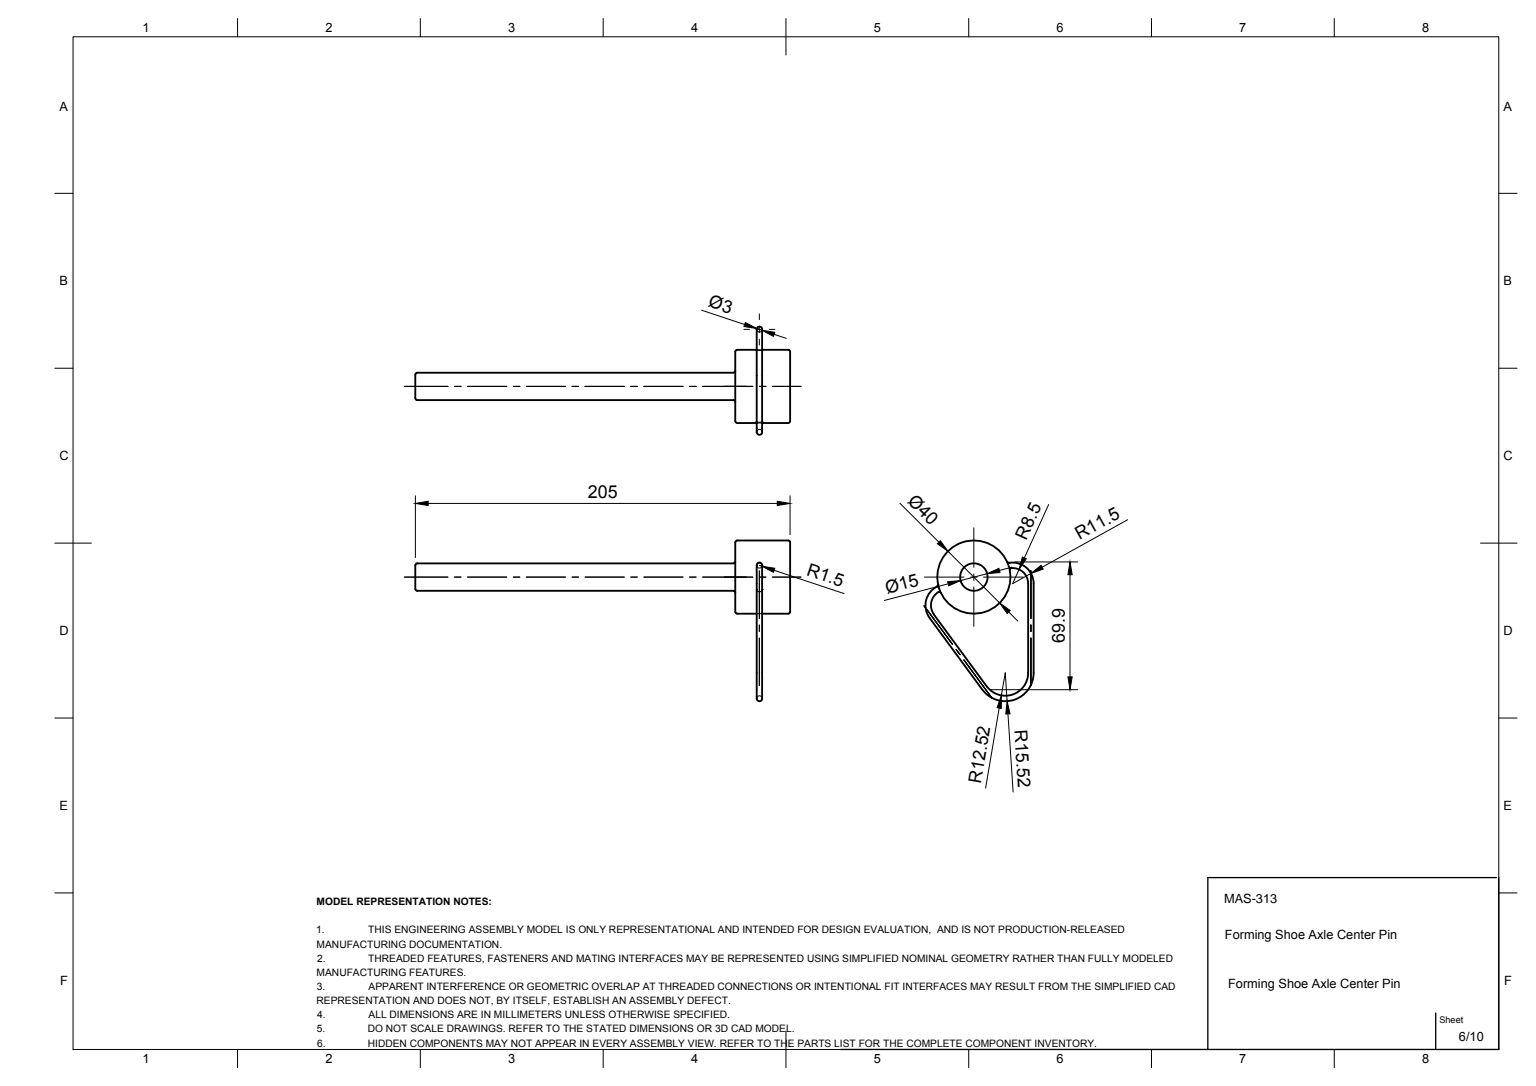
ISO-10303-21;
HEADER;
FILE_DESCRIPTION (('STEP AP214'),
    '1' );
FILE_NAME ('Forming Shoe Axle Center Pin.step',
    '2026-10-06T09:36:00',
    ( '' ),
    ( '' ),
    'SwSTEP 2.0',
    'SolidWorks 2025',
    '' );
FILE_SCHEMA (( 'AUTOMOTIVE_DESIGN' ));
ENDSEC;

DATA;
#20=VERTEX_POINT ( 'NONE', #8026 ) ;
#27=AXIS2_PLACEMENT_3D ( 'NONE', #9687, #6908, #2335 ) ;
#30=CARTESIAN_POINT ( 'NONE',  ( 19.97706055966621008, 179.9215598820742628, -126.1361639878079757 ) ) ;
#44=CARTESIAN_POINT ( 'NONE',  ( -20.77482174596512010, 180.9926187296579201, -123.5402880645762451 ) ) ;
#47=EDGE_CURVE ( 'NONE', #6610, #12185, #4189, .T. ) ;
#58=ORIENTED_EDGE ( 'NONE', *, *, #10485, .F. ) ;
#78=CARTESIAN_POINT ( 'NONE',  ( 19.99739293773369653, 178.7258229095291426, -125.0390604444466902 ) ) ;
#93=EDGE_CURVE ( 'NONE', #7054, #9028, #4139, .T. ) ;
#99=FACE_OUTER_BOUND ( 'NONE', #2484, .T. ) ;
#100=CARTESIAN_POINT ( 'NONE',  ( -19.99217429592516737, 178.8549194765174946, -125.3522826812394584 ) ) ;
#108=CARTESIAN_POINT ( 'NONE',  ( 19.97032670689476674, 177.8811654734197134, -125.7875625598146883 ) ) ;
#126=CARTESIAN_POINT ( 'NONE',  ( 19.97657209060318806, 179.2792238463859746, -123.5006916350263282 ) ) ;
#127=CARTESIAN_POINT ( 'NONE',  ( -21.00467209899894172, 181.7165653707129422, -124.9111601018296795 ) ) ;
#151=CARTESIAN_POINT ( 'NONE',  ( -19.98114923013653765, 179.3963068953591176, -125.9321215961336975 ) ) ;
#154=VERTEX_POINT ( 'NONE', #2390 ) ;
#156=AXIS2_PLACEMENT_3D ( 'NONE', #6549, #9206, #9335 ) ;
#159=DIRECTION ( 'NONE',  ( -1.186840563529527301E-16, 1.000000000000000000, -0.000000000000000000 ) ) ;
#162=CARTESIAN_POINT ( 'NONE',  ( -20.82968904857387216, 181.3053215700974192, -123.7910769712144798 ) ) ;
#176=AXIS2_PLACEMENT_3D ( 'NONE', #10566, #11560, #2167 ) ;
#213=VECTOR ( 'NONE', #11605, 1000.000000000000000 ) ;
#221=DIRECTION ( 'NONE',  ( -1.000000000000000000, 0.000000000000000000, 0.000000000000000000 ) ) ;
#222=CARTESIAN_POINT ( 'NONE',  ( 19.92179295512113057, 178.7027072646551744, -122.9085123094865537 ) ) ;
#236=DIRECTION ( 'NONE',  ( -0.000000000000000000, -1.000000000000000000, -1.757987137413040192E-14 ) ) ;
#248=FACE_OUTER_BOUND ( 'NONE', #11895, .T. ) ;
#255=CARTESIAN_POINT ( 'NONE',  ( 20.99826841500651753, 178.6919330321067036, -124.8534679218782770 ) ) ;
#262=DIRECTION ( 'NONE',  ( 1.186840563529527301E-16, -1.000000000000000000, 0.000000000000000000 ) ) ;
#274=CARTESIAN_POINT ( 'NONE',  ( -21.06063637301984670, 178.9270029669538360, -125.6999331669520501 ) ) ;
#275=CIRCLE ( 'NONE', #3413, 1.000000000000001110 ) ;
#289=ORIENTED_EDGE ( 'NONE', *, *, #5265, .F. ) ;
#292=CARTESIAN_POINT ( 'NONE',  ( -13.32222501832919193, 180.2041921146325762, -184.1652315311841051 ) ) ;
#295=CARTESIAN_POINT ( 'NONE',  ( -7.499999999999979572, -6.999999999999979572, -124.6807709998038405 ) ) ;
#303=DIRECTION ( 'NONE',  ( -1.186840563529527301E-16, 1.000000000000000000, -0.000000000000000000 ) ) ;
#307=EDGE_CURVE ( 'NONE', #1954, #154, #9065, .T. ) ;
#332=AXIS2_PLACEMENT_3D ( 'NONE', #843, #8325, #8259 ) ;
#337=CARTESIAN_POINT ( 'NONE',  ( 19.00000000000000000, 197.0000000000000000, -124.6807709998038405 ) ) ;
#372=DIRECTION ( 'NONE',  ( 0.000000000000000000, -1.000000000000000000, -1.850371707708592551E-14 ) ) ;
#377=EDGE_LOOP ( 'NONE', ( #4540, #1681, #1210, #5686, #11186, #2942, #6085, #5745, #3833, #8762 ) ) ;
#406=PRODUCT_DEFINITION ( 'UNKNOWN', '', #11578, #8636 ) ;
#416=CARTESIAN_POINT ( 'NONE',  ( 19.96510381999703654, 179.6655525025668680, -123.2864411696423019 ) ) ;
#423=AXIS2_PLACEMENT_3D ( 'NONE', #2783, #4705, #7030 ) ;
#446=ADVANCED_FACE ( 'NONE', ( #2952 ), #990, .T. ) ;
#447=ORIENTED_EDGE ( 'NONE', *, *, #3448, .T. ) ;
#457=CARTESIAN_POINT ( 'NONE',  ( -20.81528965651789420, 181.2703058956580264, -123.7202784472551258 ) ) ;
#459=CARTESIAN_POINT ( 'NONE',  ( 19.83353877203827764, 180.5116607636902302, -127.2558091114354966 ) ) ;
#460=CARTESIAN_POINT ( 'NONE',  ( 19.88442870626286307, 179.4513098237186455, -122.5333155736647655 ) ) ;
#462=VECTOR ( 'NONE', #11784, 1000.000000000000000 ) ;
#465=CARTESIAN_POINT ( 'NONE',  ( 20.00000000000000000, 197.0000000000000000, -124.6807709998038405 ) ) ;
#476=DIRECTION ( 'NONE',  ( 0.000000000000000000, 1.632680918566399772E-14, -1.000000000000000000 ) ) ;
#490=ADVANCED_FACE ( 'NONE', ( #99 ), #10651, .T. ) ;
#491=CARTESIAN_POINT ( 'NONE',  ( -20.90635653397698590, 181.5182364730088125, -122.6997973820476489 ) ) ;
#497=CARTESIAN_POINT ( 'NONE',  ( -19.97664783916611952, 180.3484222408143296, -126.1556734819005925 ) ) ;
#505=VERTEX_POINT ( 'NONE', #2202 ) ;
#513=CARTESIAN_POINT ( 'NONE',  ( -19.99999999999999645, 177.7115707886035807, -124.6807709997916334 ) ) ;
#520=CARTESIAN_POINT ( 'NONE',  ( 7.750278301654327992E-16, 197.0000000000000000, -124.6807709998038405 ) ) ;
#527=CARTESIAN_POINT ( 'NONE',  ( 19.83120603885254951, 180.1820437873792287, -127.2737130629590041 ) ) ;
#539=FACE_OUTER_BOUND ( 'NONE', #6413, .T. ) ;
#547=CARTESIAN_POINT ( 'NONE',  ( 19.96803729195536548, 180.8767316306619932, -123.3312649246138051 ) ) ;
#552=CIRCLE ( 'NONE', #6873, 0.9999999999999986677 ) ;
#556=CARTESIAN_POINT ( 'NONE',  ( 19.03136272649511085, 180.2041921146316668, -134.6807709998038547 ) ) ;
#559=VERTEX_POINT ( 'NONE', #337 ) ;
#567=CARTESIAN_POINT ( 'NONE',  ( -19.85757705203717549, 179.1763491573645979, -127.0639759997010714 ) ) ;
#569=VERTEX_POINT ( 'NONE', #9980 ) ;
#573=ORIENTED_EDGE ( 'NONE', *, *, #3270, .F. ) ;
#574=B_SPLINE_CURVE_WITH_KNOTS ( 'NONE', 3,
 ( #6859, #1412, #10623, #7851, #11679, #11625, #6974, #2280, #11742, #8936, #3144, #10680, #1355, #2218 ),
 .UNSPECIFIED., .F., .F.,
 ( 4, 2, 2, 2, 2, 2, 4 ),
 ( 0.005787645201702338975, 0.006295307287268509314, 0.006802969372834680520, 0.007818293543967111403, 0.008833617715099544021, 0.009341279800665706554, 0.009848941886231869086 ),
 .UNSPECIFIED. ) ;
#583=CARTESIAN_POINT ( 'NONE',  ( -7.500000000000004441, 197.0000000000000000, -124.6807709998038405 ) ) ;
#585=DIRECTION ( 'NONE',  ( -1.186840563529527301E-16, 1.000000000000000000, -0.000000000000000000 ) ) ;
#587=CARTESIAN_POINT ( 'NONE',  ( -21.05657978152897769, 178.8587358379057548, -125.5860039436037567 ) ) ;
#588=( NAMED_UNIT ( * ) SI_UNIT ( $, .STERADIAN. ) SOLID_ANGLE_UNIT ( ) );
#598=B_SPLINE_CURVE_WITH_KNOTS ( 'NONE', 3,
 ( #6314, #1680, #9286, #7245, #826, #4597, #888, #8437, #5439, #11267, #7428, #8371, #4716, #2601, #5375, #11011, #757, #9151, #3650, #4535 ),
 .UNSPECIFIED., .F., .F.,
 ( 4, 2, 2, 2, 2, 2, 2, 2, 2, 4 ),
 ( 0.009933187713138447172, 0.01060625352217340472, 0.01094278642669084187, 0.01127931933120827901, 0.01195238514024315329, 0.01262545094927802758, 0.01329851675831290360, 0.01397158256734777788, 0.01464464837638265217, 0.01531771418541752645 ),
 .UNSPECIFIED. ) ;
#608=CARTESIAN_POINT ( 'NONE',  ( 20.00048861043547177, 181.7193014332009113, -124.6844417253709025 ) ) ;
#610=CARTESIAN_POINT ( 'NONE',  ( 19.89275938512204078, 181.1945314693525972, -122.6057198881955941 ) ) ;
#611=AXIS2_PLACEMENT_3D ( 'NONE', #3672, #6457, #11093 ) ;
#612=CARTESIAN_POINT ( 'NONE',  ( -19.97551221440360436, 178.0138700112367758, -123.6762749394707441 ) ) ;
#616=EDGE_CURVE ( 'NONE', #4019, #1329, #9737, .T. ) ;
#618=DIRECTION ( 'NONE',  ( -0.000000000000000000, -1.000000000000000000, -1.757987137413040192E-14 ) ) ;
#630=CARTESIAN_POINT ( 'NONE',  ( -21.06735260060543879, 180.9331586078316150, -126.2486801514333905 ) ) ;
#636=DIRECTION ( 'NONE',  ( -1.186840563529527301E-16, 1.000000000000000000, -0.000000000000000000 ) ) ;
#646=CIRCLE ( 'NONE', #1249, 11.50000000000003730 ) ;
#651=EDGE_CURVE ( 'NONE', #6732, #6027, #3151, .T. ) ;
#659=CARTESIAN_POINT ( 'NONE',  ( -20.73244433232022033, 180.6366558386295935, -123.3579215951269248 ) ) ;
#674=CARTESIAN_POINT ( 'NONE',  ( 19.99815408692506580, 181.6905235212389869, -124.9672463342703566 ) ) ;
#677=CARTESIAN_POINT ( 'NONE',  ( -19.83634048512597658, 179.7265707582143079, -127.2348386560517781 ) ) ;
#692=ADVANCED_FACE ( 'NONE', ( #4300 ), #5147, .T. ) ;
#695=ORIENTED_EDGE ( 'NONE', *, *, #8586, .T. ) ;
#712=ORIENTED_EDGE ( 'NONE', *, *, #11302, .F. ) ;
#713=CARTESIAN_POINT ( 'NONE',  ( -21.06729583384051097, 179.4139655881280078, -126.1965993184190040 ) ) ;
#737=ORIENTED_EDGE ( 'NONE', *, *, #10086, .T. ) ;
#740=EDGE_CURVE ( 'NONE', #4344, #2611, #2200, .T. ) ;
#750=CARTESIAN_POINT ( 'NONE',  ( -20.00000000000000000, 197.0000000000000000, -124.6807709998038405 ) ) ;
#757=CARTESIAN_POINT ( 'NONE',  ( 19.83551131833741010, 179.7633983601342038, -127.2411838750873727 ) ) ;
#761=LINE ( 'NONE', #10215, #10128 ) ;
#765=ORIENTED_EDGE ( 'NONE', *, *, #11667, .F. ) ;
#768=CARTESIAN_POINT ( 'NONE',  ( -19.87519864879851994, 178.8871479037923393, -126.9115732480538838 ) ) ;
#770=( BOUNDED_SURFACE ( )  B_SPLINE_SURFACE ( 3, 2, ( 
 ( #7122, #2418, #6198 ),
 ( #9783, #2308, #9966 ),
 ( #6078, #8742, #659 ),
 ( #4630, #9252, #12035 ),
 ( #4435, #11044, #2570 ),
 ( #795, #4563, #923 ),
 ( #8340, #4499, #8410 ),
 ( #2770, #1648, #11178 ),
 ( #8211, #9122, #11245 ),
 ( #11973, #3548, #3689 ),
 ( #12104, #12172, #2702 ),
 ( #5409, #9317, #7337 ),
 ( #3613, #862, #7404 ),
 ( #6473, #11109, #3491 ),
 ( #7276, #6341, #10116 ),
 ( #10247, #2631, #1842 ),
 ( #6410, #1782, #7465 ),
 ( #5545, #6534, #10302 ),
 ( #5606, #9383, #4696 ),
 ( #10608, #11354, #7646 ),
 ( #3810, #10544, #8576 ),
 ( #9441, #10489, #4918 ),
 ( #8700, #100, #978 ),
 ( #3874, #9680, #9559 ),
 ( #7582, #2953, #274 ),
 ( #3998, #6715, #2022 ),
 ( #1105, #1218, #8639 ),
 ( #5911, #2146, #2091 ),
 ( #8758, #151, #9619 ),
 ( #7766, #4065, #5460 ) ),
 .UNSPECIFIED., .F., .F., .F. ) 
 B_SPLINE_SURFACE_WITH_KNOTS ( ( 4, 2, 2, 2, 2, 2, 2, 2, 2, 2, 2, 2, 2, 2, 4 ),
 ( 3, 3 ),
 ( 0.007888614278243437361, 0.008874691063023869633, 0.009367729455414086637, 0.009860767847804301905, 0.01035380624019451891, 0.01084684463258473591, 0.01133988302497495118, 0.01183292141736516818, 0.01281899820214560046, 0.01331203659453581746, 0.01380507498692603446, 0.01429811337931624973, 0.01479115177170646674, 0.01528419016409668374, 0.01577722855648689901 ),
 ( 0.000000000000000000, 1.000000000000000000 ),
 .UNSPECIFIED. ) 
 GEOMETRIC_REPRESENTATION_ITEM ( )  RATIONAL_B_SPLINE_SURFACE ( (
 ( 1.000000000000000000, 0.7778924984312529656, 1.000000000000000000),
 ( 1.000000000000000000, 0.7847112435279847142, 1.000000000000000000),
 ( 1.000000000000000000, 0.7894485421771765266, 1.000000000000000000),
 ( 1.000000000000000000, 0.7926414855251958658, 1.000000000000000000),
 ( 1.000000000000000000, 0.7930469064958857173, 1.000000000000000000),
 ( 1.000000000000000000, 0.7925074991235926403, 1.000000000000000000),
 ( 1.000000000000000000, 0.7915770372355392936, 1.000000000000000000),
 ( 1.000000000000000000, 0.7883898363194743464, 1.000000000000000000),
 ( 1.000000000000000000, 0.7861853387937841608, 1.000000000000000000),
 ( 1.000000000000000000, 0.7806815604416567078, 1.000000000000000000),
 ( 1.000000000000000000, 0.7773361016722152295, 1.000000000000000000),
 ( 1.000000000000000000, 0.7698701636707948603, 1.000000000000000000),
 ( 1.000000000000000000, 0.7657526702509508398, 1.000000000000000000),
 ( 1.000000000000000000, 0.7568812398704235500, 1.000000000000000000),
 ( 1.000000000000000000, 0.7521322257284934754, 1.000000000000000000),
 ( 1.000000000000000000, 0.7377220824064392168, 1.000000000000000000),
 ( 1.000000000000000000, 0.7275566802060602356, 1.000000000000000000),
 ( 1.000000000000000000, 0.7135779984947178134, 1.000000000000000000),
 ( 1.000000000000000000, 0.7090467312072497030, 1.000000000000000000),
 ( 1.000000000000000000, 0.7006183237057392876, 1.000000000000000000),
 ( 1.000000000000000000, 0.6967528866742972449, 1.000000000000000000),
 ( 1.000000000000000000, 0.6897151435478420245, 1.000000000000000000),
 ( 1.000000000000000000, 0.6865208713865151857, 1.000000000000000000),
 ( 1.000000000000000000, 0.6810351634549236532, 1.000000000000000000),
 ( 1.000000000000000000, 0.6787116622188523740, 1.000000000000000000),
 ( 1.000000000000000000, 0.6747765002012137137, 1.000000000000000000),
 ( 1.000000000000000000, 0.6731806124592021323, 1.000000000000000000),
 ( 1.000000000000000000, 0.6706618708365198467, 1.000000000000000000),
 ( 1.000000000000000000, 0.6697163794380122104, 1.000000000000000000),
 ( 1.000000000000000000, 0.6689879873414465994, 1.000000000000000000) ) ) 
 REPRESENTATION_ITEM ( '' )  SURFACE ( )  );
#773=CARTESIAN_POINT ( 'NONE',  ( 19.87268743161337170, 178.9255784920988503, -126.9338343023757290 ) ) ;
#780=ORIENTED_EDGE ( 'NONE', *, *, #4037, .T. ) ;
#786=DIRECTION ( 'NONE',  ( -1.000000000000000000, 0.000000000000000000, 0.000000000000000000 ) ) ;
#791=CIRCLE ( 'NONE', #11439, 12.52076803445814690 ) ;
#792=PLANE ( 'NONE',  #6380 ) ;
#795=CARTESIAN_POINT ( 'NONE',  ( -19.87376422533415266, 179.9397883299151601, -122.4372163154974942 ) ) ;
#804=CARTESIAN_POINT ( 'NONE',  ( 21.06240745282767435, 180.2041921146315246, -126.4269926335259413 ) ) ;
#808=CARTESIAN_POINT ( 'NONE',  ( 19.86936981681406778, 181.4590435457396609, -126.9708661016945257 ) ) ;
#822=VERTEX_POINT ( 'NONE', #12019 ) ;
#826=CARTESIAN_POINT ( 'NONE',  ( 19.98066683771208574, 182.6001984525962030, -125.5662099944124748 ) ) ;
#830=CARTESIAN_POINT ( 'NONE',  ( -19.99331759212207515, 182.5955720455716573, -124.1413515841623649 ) ) ;
#839=AXIS2_PLACEMENT_3D ( 'NONE', #11119, #4323, #8349 ) ;
#843=CARTESIAN_POINT ( 'NONE',  ( -19.03136272649511085, 180.2041921146316668, -134.6807709998038547 ) ) ;
#862=CARTESIAN_POINT ( 'NONE',  ( -19.98517529853678809, 179.0632710820790976, -123.7013734869633197 ) ) ;
#870=CARTESIAN_POINT ( 'NONE',  ( 19.99218703114167539, 182.5822718396941582, -124.1010742661679274 ) ) ;
#888=CARTESIAN_POINT ( 'NONE',  ( 19.96426536123311735, 182.4767232793243181, -125.8798892712007245 ) ) ;
#894=CARTESIAN_POINT ( 'NONE',  ( -20.00092085174054546, 181.7296212712162173, -124.7139161294905136 ) ) ;
#909=CARTESIAN_POINT ( 'NONE',  ( 21.04869859328100290, 178.8069441414488097, -125.4530315734257471 ) ) ;
#913=EDGE_CURVE ( 'NONE', #9220, #9416, #3010, .T. ) ;
#914=AXIS2_PLACEMENT_3D ( 'NONE', #2500, #4427, #1515 ) ;
#923=CARTESIAN_POINT ( 'NONE',  ( -20.72096896666972299, 180.0455498438134896, -123.3107784691637079 ) ) ;
#926=CARTESIAN_POINT ( 'NONE',  ( -21.06240745282767080, 180.2041921146517041, -126.4269926335259413 ) ) ;
#927=ORIENTED_EDGE ( 'NONE', *, *, #5402, .T. ) ;
#936=DIRECTION ( 'NONE',  ( -0.000000000000000000, -1.000000000000000000, -1.757987137413040192E-14 ) ) ;
#942=EDGE_LOOP ( 'NONE', ( #4491, #737, #7354, #4686, #5672 ) ) ;
#955=B_SPLINE_CURVE_WITH_KNOTS ( 'NONE', 3,
 ( #11864, #5021, #2525, #4106, #10938, #8230, #9138, #11926, #3379, #10652, #7171, #10998, #5360, #612, #1542, #5303, #3167, #6016 ),
 .UNSPECIFIED., .F., .F.,
 ( 4, 2, 2, 2, 2, 2, 2, 2, 4 ),
 ( 0.007924218878882885106, 0.008564103707084826447, 0.009203988535286766054, 0.009843873363488707395, 0.01048375819169064874, 0.01112364301989258834, 0.01176352784809452968, 0.01240341267629646929, 0.01304329750449841063 ),
 .UNSPECIFIED. ) ;
#968=CARTESIAN_POINT ( 'NONE',  ( 27.10787553788151172, 180.2041921146317520, -137.3302880892914288 ) ) ;
#971=ORIENTED_EDGE ( 'NONE', *, *, #9425, .T. ) ;
#978=CARTESIAN_POINT ( 'NONE',  ( -21.04715153834148467, 178.7974658297258372, -125.4275705862621066 ) ) ;
#980=ORIENTED_EDGE ( 'NONE', *, *, #11838, .T. ) ;
#983=AXIS2_PLACEMENT_3D ( 'NONE', #1406, #8087, #9811 ) ;
#990=TOROIDAL_SURFACE ( 'NONE', #6899, 10.00000000000002487, 1.499999999999998002 ) ;
#1006=CARTESIAN_POINT ( 'NONE',  ( 20.86846003075320866, 178.9597637446144631, -123.9944097082106396 ) ) ;
#1007=EDGE_CURVE ( 'NONE', #6027, #2717, #3007, .T. ) ;
#1009=CARTESIAN_POINT ( 'NONE',  ( -20.00222207760924320, 182.7106143631367559, -124.6033207595390593 ) ) ;
#1015=FACE_OUTER_BOUND ( 'NONE', #7771, .T. ) ;
#1028=ORIENTED_EDGE ( 'NONE', *, *, #10086, .F. ) ;
#1036=EDGE_CURVE ( 'NONE', #7665, #6732, #955, .T. ) ;
#1039=FACE_OUTER_BOUND ( 'NONE', #11944, .T. ) ;
#1040=CARTESIAN_POINT ( 'NONE',  ( 21.06408185580648862, 179.7982817377094591, -126.3732375885690260 ) ) ;
#1052=CARTESIAN_POINT ( 'NONE',  ( -19.03136272649511085, 180.2041921146316668, -134.6807709998038547 ) ) ;
#1054=CARTESIAN_POINT ( 'NONE',  ( 19.94460181908782914, 178.0949482486194597, -126.1813690857228636 ) ) ;
#1057=EDGE_LOOP ( 'NONE', ( #6785, #9431, #1351, #2666, #10669 ) ) ;
#1059=DIRECTION ( 'NONE',  ( -0.3117078928809425831, -5.319854888938806247E-14, 0.9501779778103273122 ) ) ;
#1071=CARTESIAN_POINT ( 'NONE',  ( 19.96762839730446260, 179.5630691651248299, -123.3296266449212766 ) ) ;
#1085=EDGE_LOOP ( 'NONE', ( #10428, #11076, #8480, #3695 ) ) ;
#1105=CARTESIAN_POINT ( 'NONE',  ( -19.91567555516949994, 178.3764997479877650, -126.5185459719826468 ) ) ;
#1106=CARTESIAN_POINT ( 'NONE',  ( 19.03136272649511085, 180.2041921146316668, -134.6807709998038547 ) ) ;
#1126=PRODUCT_DEFINITION_SHAPE ( 'NONE', 'NONE',  #406 ) ;
#1161=FACE_OUTER_BOUND ( 'NONE', #10213, .T. ) ;
#1162=AXIS2_PLACEMENT_3D ( 'NONE', #4182, #1345, #5107 ) ;
#1172=CIRCLE ( 'NONE', #8067, 1.500000000000001332 ) ;
#1187=EDGE_CURVE ( 'NONE', #3899, #2611, #5763, .T. ) ;
#1202=EDGE_LOOP ( 'NONE', ( #3605, #10463 ) ) ;
#1206=CARTESIAN_POINT ( 'NONE',  ( -19.99999999999992184, 182.7057073811386658, -124.7928861707884494 ) ) ;
#1210=ORIENTED_EDGE ( 'NONE', *, *, #1523, .T. ) ;
#1218=CARTESIAN_POINT ( 'NONE',  ( -19.98421530564996473, 179.1834412406901151, -125.7728037431097619 ) ) ;
#1249=AXIS2_PLACEMENT_3D ( 'NONE', #8612, #6689, #6811 ) ;
#1258=EDGE_CURVE ( 'NONE', #4474, #4344, #12188, .T. ) ;
#1261=CARTESIAN_POINT ( 'NONE',  ( -19.99234306063619471, 182.6762740227041206, -125.2450393957101653 ) ) ;
#1283=ORIENTED_EDGE ( 'NONE', *, *, #5915, .F. ) ;
#1299=CIRCLE ( 'NONE', #5225, 19.00000000000000000 ) ;
#1310=CARTESIAN_POINT ( 'NONE',  ( 19.97422267005788044, 181.0592659262004247, -123.4551364493781733 ) ) ;
#1322=CARTESIAN_POINT ( 'NONE',  ( -19.85981914806637860, 181.2821069731401735, -127.0472120087121652 ) ) ;
#1323=FACE_OUTER_BOUND ( 'NONE', #10059, .T. ) ;
#1329=VERTEX_POINT ( 'NONE', #10442 ) ;
#1345=DIRECTION ( 'NONE',  ( 0.3117078928809249860, 1.670400663243698742E-14, -0.9501779778103330854 ) ) ;
#1348=CARTESIAN_POINT ( 'NONE',  ( 19.94418390071693281, 178.3880804771991677, -123.1813497959713004 ) ) ;
#1351=ORIENTED_EDGE ( 'NONE', *, *, #11667, .T. ) ;
#1355=CARTESIAN_POINT ( 'NONE',  ( 21.06813109674855156, 179.2925129078113571, -126.1227452162743674 ) ) ;
#1378=CARTESIAN_POINT ( 'NONE',  ( 20.91518010789754456, 178.8209456716285501, -124.2613132543053638 ) ) ;
#1381=ORIENTED_EDGE ( 'NONE', *, *, #2835, .T. ) ;
#1387=UNCERTAINTY_MEASURE_WITH_UNIT (LENGTH_MEASURE( 1.000000000000000082E-05 ), #8332, 'distance_accuracy_value', 'NONE');
#1397=LINE ( 'NONE', #4245, #462 ) ;
#1406=CARTESIAN_POINT ( 'NONE',  ( 28.53314250459842327, 180.2041921146317236, -137.7978499286132319 ) ) ;
#1412=CARTESIAN_POINT ( 'NONE',  ( 20.71964524312697620, 180.0370539397483185, -123.3053720114571519 ) ) ;
#1413=DIRECTION ( 'NONE',  ( -1.000000000000000000, 0.000000000000000000, 0.000000000000000000 ) ) ;
#1419=CARTESIAN_POINT ( 'NONE',  ( -19.03136272649511085, 180.2041921146316668, -134.6807709998038547 ) ) ;
#1428=DIRECTION ( 'NONE',  ( -1.000000000000000000, 0.000000000000000000, 0.000000000000000000 ) ) ;
#1430=DIRECTION ( 'NONE',  ( -1.000000000000000000, 0.000000000000000000, 0.000000000000000000 ) ) ;
#1448=FACE_OUTER_BOUND ( 'NONE', #11473, .T. ) ;
#1453=CIRCLE ( 'NONE', #4229, 1.500000000000001332 ) ;
#1482=EDGE_LOOP ( 'NONE', ( #2546, #3392, #12236, #9462 ) ) ;
#1498=FACE_OUTER_BOUND ( 'NONE', #3824, .T. ) ;
#1515=DIRECTION ( 'NONE',  ( -1.000000000000000000, 0.000000000000000000, 0.000000000000000000 ) ) ;
#1516=ORIENTED_EDGE ( 'NONE', *, *, #5402, .F. ) ;
#1520=CARTESIAN_POINT ( 'NONE',  ( 19.90865200055593220, 181.4799304009739558, -122.7714319726113104 ) ) ;
#1523=EDGE_CURVE ( 'NONE', #2536, #6732, #761, .T. ) ;
#1541=ADVANCED_FACE ( 'NONE', ( #1498 ), #4158, .F. ) ;
#1542=CARTESIAN_POINT ( 'NONE',  ( -19.98431733801637122, 177.9165942756023640, -123.8639317673912785 ) ) ;
#1543=DIRECTION ( 'NONE',  ( 1.000000000000000000, 1.186840563529527301E-16, 0.000000000000000000 ) ) ;
#1555=CARTESIAN_POINT ( 'NONE',  ( -19.97950307607502296, 180.8737719992032567, -126.0168746971561688 ) ) ;
#1556=DIRECTION ( 'NONE',  ( -0.000000000000000000, -1.000000000000000000, -1.757987137413040192E-14 ) ) ;
#1596=CARTESIAN_POINT ( 'NONE',  ( 19.98721147511798080, 181.3928720024498205, -123.7411646176790327 ) ) ;
#1620=CARTESIAN_POINT ( 'NONE',  ( -19.97661686088444810, 180.0768701897325741, -126.1571822173844453 ) ) ;
#1627=CIRCLE ( 'NONE', #5771, 7.500000000000005329 ) ;
#1645=EDGE_CURVE ( 'NONE', #8550, #1954, #6674, .T. ) ;
#1648=CARTESIAN_POINT ( 'NONE',  ( -19.96447914003645607, 179.6944185909774490, -123.2758706440192213 ) ) ;
#1651=ORIENTED_EDGE ( 'NONE', *, *, #3988, .F. ) ;
#1661=CARTESIAN_POINT ( 'NONE',  ( 19.99452644844618732, 181.5558364952455577, -124.0087194824425865 ) ) ;
#1671=AXIS2_PLACEMENT_3D ( 'NONE', #8007, #9792, #8865 ) ;
#1680=CARTESIAN_POINT ( 'NONE',  ( 19.99999999999986855, 182.7144438187336277, -124.9030158930556667 ) ) ;
#1681=ORIENTED_EDGE ( 'NONE', *, *, #11312, .T. ) ;
#1692=EDGE_CURVE ( 'NONE', #11672, #7759, #8013, .T. ) ;
#1693=CYLINDRICAL_SURFACE ( 'NONE', #8004, 1.500000000000000444 ) ;
#1695=CARTESIAN_POINT ( 'NONE',  ( 21.06714599819344258, 179.1261101450867557, -125.9628648169738625 ) ) ;
#1714=CARTESIAN_POINT ( 'NONE',  ( 19.86348653241994100, 179.0685786869776450, -127.0149889656965740 ) ) ;
#1728=FACE_BOUND ( 'NONE', #8840, .T. ) ;
#1731=CARTESIAN_POINT ( 'NONE',  ( 19.92971727147881467, 178.2306503425758990, -126.3637072540984292 ) ) ;
#1733=CARTESIAN_POINT ( 'NONE',  ( 20.00016885954969226, 181.6903612530189491, -124.3916023546908463 ) ) ;
#1739=CARTESIAN_POINT ( 'NONE',  ( 21.06635469844951558, 179.5529625613920643, -126.2817468820535964 ) ) ;
#1745=TOROIDAL_SURFACE ( 'NONE', #10019, 6.500000000000005329, 1.000000000000000000 ) ;
#1774=DIRECTION ( 'NONE',  ( -1.186840563529527301E-16, 1.000000000000000000, -0.000000000000000000 ) ) ;
#1782=CARTESIAN_POINT ( 'NONE',  ( -20.00091651665146841, 178.6995461844927888, -124.4414934301431401 ) ) ;
#1784=ORIENTED_EDGE ( 'NONE', *, *, #8193, .F. ) ;
#1791=CARTESIAN_POINT ( 'NONE',  ( 19.96940092271958278, 182.5175105289615942, -125.7966324820120008 ) ) ;
#1803=ORIENTED_EDGE ( 'NONE', *, *, #8190, .F. ) ;
#1814=CARTESIAN_POINT ( 'NONE',  ( -19.99532149354086030, 181.6339454046986361, -125.1698373029890519 ) ) ;
#1815=DIRECTION ( 'NONE',  ( 0.3117078928809249860, 1.670400663243698742E-14, -0.9501779778103330854 ) ) ;
#1824=TOROIDAL_SURFACE ( 'NONE', #10885, 10.00000000000002487, 1.499999999999998002 ) ;
#1826=CARTESIAN_POINT ( 'NONE',  ( 19.99178670042469719, 178.8663240180210039, -125.3736306701222532 ) ) ;
#1841=DIRECTION ( 'NONE',  ( -0.000000000000000000, -1.000000000000000000, -1.757987137413040192E-14 ) ) ;
#1842=CARTESIAN_POINT ( 'NONE',  ( -20.91120072986939959, 178.8231192296793779, -124.2317959954639406 ) ) ;
#1852=ADVANCED_FACE ( 'NONE', ( #9118 ), #792, .F. ) ;
#1853=CARTESIAN_POINT ( 'NONE',  ( 21.06610394755309201, 181.3758997718305181, -125.8629927389160486 ) ) ;
#1854=CARTESIAN_POINT ( 'NONE',  ( 19.98052438014507715, 181.2452332506350672, -123.5813376981535043 ) ) ;
#1858=DIRECTION ( 'NONE',  ( -0.9501779778103373042, 0.000000000000000000, 0.3117078928809121074 ) ) ;
#1876=CARTESIAN_POINT ( 'NONE',  ( -20.87666491430435300, 181.4765249126461129, -124.0391332007959306 ) ) ;
#1893=MECHANICAL_DESIGN_GEOMETRIC_PRESENTATION_REPRESENTATION('',(#3255),#10179);
#1898=EDGE_LOOP ( 'NONE', ( #2480, #3346, #2420, #11357 ) ) ;
#1904=CARTESIAN_POINT ( 'NONE',  ( -6.499999999999979572, -7.999999999999979572, -124.6807709998038405 ) ) ;
#1911=ADVANCED_FACE ( 'NONE', ( #1039 ), #3814, .T. ) ;
#1912=CARTESIAN_POINT ( 'NONE',  ( -19.92695522958598175, 181.7999794737119430, -122.9644587262777549 ) ) ;
#1934=CARTESIAN_POINT ( 'NONE',  ( -19.93883021351429363, 182.2592841156773602, -126.2495949291102022 ) ) ;
#1954=VERTEX_POINT ( 'NONE', #926 ) ;
#1978=CARTESIAN_POINT ( 'NONE',  ( 20.96631641705466365, 181.6890404706723530, -124.5993264551280646 ) ) ;
#1993=CARTESIAN_POINT ( 'NONE',  ( 20.76787417662263735, 179.4594239414511492, -123.5091856982008949 ) ) ;
#1995=CARTESIAN_POINT ( 'NONE',  ( -20.00032812729986631, 181.6954111208232518, -124.4177824055624058 ) ) ;
#2016=AXIS2_PLACEMENT_3D ( 'NONE', #1419, #8941, #476 ) ;
#2022=CARTESIAN_POINT ( 'NONE',  ( -21.06555081338637692, 179.0416688902717510, -125.8654226178028068 ) ) ;
#2048=EDGE_LOOP ( 'NONE', ( #3175, #9799 ) ) ;
#2049=CARTESIAN_POINT ( 'NONE',  ( 20.85245725203401079, 179.0178972154230621, -123.9104686020650519 ) ) ;
#2058=CARTESIAN_POINT ( 'NONE',  ( -30.53136272649514638, 180.2041921146316668, -134.6807709998038547 ) ) ;
#2066=AXIS2_PLACEMENT_3D ( 'NONE', #10321, #3831, #9518 ) ;
#2080=AXIS2_PLACEMENT_3D ( 'NONE', #6022, #262, #4051 ) ;
#2091=CARTESIAN_POINT ( 'NONE',  ( -21.06800052547805535, 179.2509983577178616, -126.0809827838107964 ) ) ;
#2100=ORIENTED_EDGE ( 'NONE', *, *, #3197, .T. ) ;
#2118=ORIENTED_EDGE ( 'NONE', *, *, #12020, .T. ) ;
#2129=CARTESIAN_POINT ( 'NONE',  ( 21.01976670805043312, 178.7020268087202055, -125.0612880804587093 ) ) ;
#2139=VERTEX_POINT ( 'NONE', #1904 ) ;
#2146=CARTESIAN_POINT ( 'NONE',  ( -19.98209572305366422, 179.3222604960775186, -125.8830796407651036 ) ) ;
#2156=CARTESIAN_POINT ( 'NONE',  ( 19.00000000000000355, 168.0000000000000000, -124.6807709998038405 ) ) ;
#2157=VECTOR ( 'NONE', #11936, 1000.000000000000000 ) ;
#2167=DIRECTION ( 'NONE',  ( -0.9501779778103371932, 0.000000000000000000, 0.3117078928809124960 ) ) ;
#2181=CARTESIAN_POINT ( 'NONE',  ( -27.10787553788296833, 180.2041921146317236, -137.3302880892916846 ) ) ;
#2185=ADVANCED_FACE ( 'NONE', ( #1448 ), #10920, .T. ) ;
#2189=CARTESIAN_POINT ( 'NONE',  ( -19.84927175247429432, 181.0689383095263167, -127.1322084511289034 ) ) ;
#2200=CIRCLE ( 'NONE', #611, 15.52076803445812203 ) ;
#2202=CARTESIAN_POINT ( 'NONE',  ( 21.06714545844871367, 179.4370239411119030, -126.2109676220344596 ) ) ;
#2204=CARTESIAN_POINT ( 'NONE',  ( 2.498657532616778856E-14, -6.999999999999978684, -124.6807709998038405 ) ) ;
#2218=CARTESIAN_POINT ( 'NONE',  ( 21.06714545844871367, 179.4370239411119030, -126.2109676220344596 ) ) ;
#2249=ADVANCED_FACE ( 'NONE', ( #10903 ), #7018, .T. ) ;
#2257=AXIS2_PLACEMENT_3D ( 'NONE', #1106, #1556, #5321 ) ;
#2260=B_SPLINE_CURVE_WITH_KNOTS ( 'NONE', 3,
 ( #4171, #8188, #6030, #5204, #5266, #3349 ),
 .UNSPECIFIED., .F., .F.,
 ( 4, 2, 4 ),
 ( 0.008741033683305053648, 0.009157775081816015711, 0.009574516480326976040 ),
 .UNSPECIFIED. ) ;
#2270=CARTESIAN_POINT ( 'NONE',  ( 19.98635603549800521, 182.5149518089054652, -123.9190205516158159 ) ) ;
#2280=CARTESIAN_POINT ( 'NONE',  ( 20.99327390029534968, 178.6730123709782845, -124.7865744064447995 ) ) ;
#2287=CARTESIAN_POINT ( 'NONE',  ( -19.03136272649511085, 180.2041921146316668, -134.6807709998038547 ) ) ;
#2294=FACE_OUTER_BOUND ( 'NONE', #377, .T. ) ;
#2308=CARTESIAN_POINT ( 'NONE',  ( -19.96884611294068179, 180.9047917079184344, -123.3454246131005050 ) ) ;
#2325=CARTESIAN_POINT ( 'NONE',  ( -19.93162290699157779, 178.2126347188217608, -126.3409196197182780 ) ) ;
#2334=CARTESIAN_POINT ( 'NONE',  ( 19.97697870131679920, 180.4645185616454910, -126.1401451060182382 ) ) ;
#2335=DIRECTION ( 'NONE',  ( 0.9501779778103252028, 0.000000000000000000, 0.3117078928809489669 ) ) ;
#2350=AXIS2_PLACEMENT_3D ( 'NONE', #12130, #4765, #3955 ) ;
#2367=CARTESIAN_POINT ( 'NONE',  ( 20.94507493758783312, 178.7564165339132103, -124.4539389338348911 ) ) ;
#2368=EDGE_CURVE ( 'NONE', #4474, #3651, #4632, .T. ) ;
#2377=CARTESIAN_POINT ( 'NONE',  ( -19.90245853136579868, 178.5200732004545898, -126.6601217908411314 ) ) ;
#2381=ADVANCED_FACE ( 'NONE', ( #3596 ), #8362, .F. ) ;
#2382=( LENGTH_UNIT ( ) NAMED_UNIT ( * ) SI_UNIT ( .MILLI., .METRE. ) );
#2390=CARTESIAN_POINT ( 'NONE',  ( -27.53136272649514993, 180.2041921146316099, -134.6807709998038547 ) ) ;
#2399=CARTESIAN_POINT ( 'NONE',  ( -8.500000000000000000, 167.0000000000000000, -124.6807709998038405 ) ) ;
#2403=ORIENTED_EDGE ( 'NONE', *, *, #2933, .T. ) ;
#2404=CARTESIAN_POINT ( 'NONE',  ( 20.71987187177683509, 180.3155698455967979, -123.3062602373065175 ) ) ;
#2415=ORIENTED_EDGE ( 'NONE', *, *, #5296, .F. ) ;
#2417=CARTESIAN_POINT ( 'NONE',  ( -21.06257444491743414, 180.3615573004741464, -126.4218899470852762 ) ) ;
#2418=CARTESIAN_POINT ( 'NONE',  ( -19.97506881502268428, 181.0839254472395510, -123.4722291287969114 ) ) ;
#2420=ORIENTED_EDGE ( 'NONE', *, *, #9087, .T. ) ;
#2445=CARTESIAN_POINT ( 'NONE',  ( -21.06773542571745139, 180.9985192952500199, -126.2048741678526937 ) ) ;
#2446=AXIS2_PLACEMENT_3D ( 'NONE', #9750, #11794, #6910 ) ;
#2452=CARTESIAN_POINT ( 'NONE',  ( -19.96162039375556674, 182.2324071300824642, -123.4314723458560081 ) ) ;
#2467=CARTESIAN_POINT ( 'NONE',  ( 19.96002121859434553, 179.9932536262492135, -123.2030480363463028 ) ) ;
#2474=DIRECTION ( 'NONE',  ( 0.000000000000000000, 1.632680918566399772E-14, -1.000000000000000000 ) ) ;
#2479=CIRCLE ( 'NONE', #9785, 6.500000000000005329 ) ;
#2480=ORIENTED_EDGE ( 'NONE', *, *, #5946, .F. ) ;
#2482=CARTESIAN_POINT ( 'NONE',  ( 19.99771933579459926, 178.7804467691931052, -124.1722115321708628 ) ) ;
#2483=CARTESIAN_POINT ( 'NONE',  ( -21.06305143384230760, 180.4613526592487176, -126.4076700800818287 ) ) ;
#2484=EDGE_LOOP ( 'NONE', ( #12232, #10611, #7447, #9409 ) ) ;
#2499=DIRECTION ( 'NONE',  ( 1.000000000000000000, 0.000000000000000000, 0.000000000000000000 ) ) ;
#2500=CARTESIAN_POINT ( 'NONE',  ( -18.99999999999999645, 168.0000000000000000, -124.6807709998038405 ) ) ;
#2507=CARTESIAN_POINT ( 'NONE',  ( -21.06240745282773474, 180.3699811770686949, -126.4269926335236676 ) ) ;
#2521=CARTESIAN_POINT ( 'NONE',  ( 19.98597855131029988, 181.3192703522229863, -125.6808798714440343 ) ) ;
#2524=AXIS2_PLACEMENT_3D ( 'NONE', #9806, #4310, #10509 ) ;
#2525=CARTESIAN_POINT ( 'NONE',  ( -19.89130973751302989, 181.1405932345318206, -122.5976180991194155 ) ) ;
#2529=CIRCLE ( 'NONE', #10245, 19.00000000000000000 ) ;
#2536=VERTEX_POINT ( 'NONE', #2906 ) ;
#2545=CARTESIAN_POINT ( 'NONE',  ( -19.83130628892425307, 180.1366617011883307, -127.2729378191562120 ) ) ;
#2546=ORIENTED_EDGE ( 'NONE', *, *, #11954, .F. ) ;
#2551=CARTESIAN_POINT ( 'NONE',  ( 2.498657532616778856E-14, -6.999999999999978684, -124.6807709998038405 ) ) ;
#2552=EDGE_CURVE ( 'NONE', #822, #1329, #8388, .T. ) ;
#2570=CARTESIAN_POINT ( 'NONE',  ( -20.71893962830172953, 180.2427088464574183, -123.3024896548053988 ) ) ;
#2576=FACE_OUTER_BOUND ( 'NONE', #4132, .T. ) ;
#2580=CARTESIAN_POINT ( 'NONE',  ( 2.510525938252074008E-14, -7.999999999999979572, -124.6807709998038405 ) ) ;
#2582=CARTESIAN_POINT ( 'NONE',  ( 21.00015071161585212, 181.7073031029140679, -124.8819044078220060 ) ) ;
#2584=ORIENTED_EDGE ( 'NONE', *, *, #616, .F. ) ;
#2590=EDGE_CURVE ( 'NONE', #2717, #7665, #7502, .T. ) ;
#2598=EDGE_LOOP ( 'NONE', ( #12179, #695, #2648, #7263 ) ) ;
#2601=CARTESIAN_POINT ( 'NONE',  ( 19.83591177254676907, 180.6622834474515003, -127.2381046240775646 ) ) ;
#2611=VERTEX_POINT ( 'NONE', #4631 ) ;
#2631=CARTESIAN_POINT ( 'NONE',  ( -19.99929956756464478, 178.7451710997399346, -124.2412955515236490 ) ) ;
#2647=CARTESIAN_POINT ( 'NONE',  ( 19.89942126619322238, 181.8500073156368160, -126.6862962162580430 ) ) ;
#2648=ORIENTED_EDGE ( 'NONE', *, *, #11838, .F. ) ;
#2666=ORIENTED_EDGE ( 'NONE', *, *, #5247, .T. ) ;
#2670=CARTESIAN_POINT ( 'NONE',  ( -19.97875451785945700, 179.6374628416406836, -126.0536791248172648 ) ) ;
#2682=CARTESIAN_POINT ( 'NONE',  ( 19.92363529031039704, 178.2952318472436843, -126.4314419646907766 ) ) ;
#2700=ADVANCED_FACE ( 'NONE', ( #10303 ), #10147, .T. ) ;
#2702=CARTESIAN_POINT ( 'NONE',  ( -20.77690287681668480, 179.3967289902496134, -123.5488579070389790 ) ) ;
#2705=EDGE_LOOP ( 'NONE', ( #11668, #3001, #2118, #8690 ) ) ;
#2713=CARTESIAN_POINT ( 'NONE',  ( 21.03739706409710308, 181.6552966610061333, -125.2847076232827277 ) ) ;
#2717=VERTEX_POINT ( 'NONE', #6411 ) ;
#2719=DIRECTION ( 'NONE',  ( 0.3117078928809249860, 1.670400663243698742E-14, -0.9501779778103330854 ) ) ;
#2737=CARTESIAN_POINT ( 'NONE',  ( -21.05155671971371945, 181.5816570678630058, -125.5021982045221023 ) ) ;
#2747=EDGE_CURVE ( 'NONE', #4517, #11672, #275, .T. ) ;
#2749=CARTESIAN_POINT ( 'NONE',  ( 19.95397453693550816, 178.0155092113254227, -126.0442809803723492 ) ) ;
#2753=CLOSED_SHELL ( 'NONE', ( #1911, #692, #446, #10635, #6145, #7798, #3072, #2700, #10898, #5576, #7681, #4206, #5538, #2249, #10033, #6300, #1852, #5079, #9343, #7282, #4928, #490, #11046, #3350, #6102, #2381, #1541, #7726, #5839, #2185, #6751 ) ) ;
#2770=CARTESIAN_POINT ( 'NONE',  ( -19.88472492139865722, 179.4532041746028881, -122.5361950424904620 ) ) ;
#2771=DIRECTION ( 'NONE',  ( -1.186840563529527301E-16, 1.000000000000000000, -0.000000000000000000 ) ) ;
#2779=CARTESIAN_POINT ( 'NONE',  ( 19.98997306493104986, 181.4837338438134395, -125.4713928613115144 ) ) ;
#2780=VERTEX_POINT ( 'NONE', #11292 ) ;
#2783=CARTESIAN_POINT ( 'NONE',  ( 13.32222501832767847, 180.2041921146325762, -184.1652315311843893 ) ) ;
#2799=CARTESIAN_POINT ( 'NONE',  ( -19.98689171310115853, 181.3620631069858007, -125.6334417695027525 ) ) ;
#2809=CARTESIAN_POINT ( 'NONE',  ( 21.06773055716234211, 179.3512387574996012, -126.1585967055013100 ) ) ;
#2815=TOROIDAL_SURFACE ( 'NONE', #9720, 19.00000000000000000, 1.000000000000000000 ) ;
#2816=ORIENTED_EDGE ( 'NONE', *, *, #8640, .T. ) ;
#2835=EDGE_CURVE ( 'NONE', #9028, #7759, #11544, .T. ) ;
#2837=EDGE_CURVE ( 'NONE', #559, #9851, #5396, .T. ) ;
#2841=CARTESIAN_POINT ( 'NONE',  ( 21.05611512818808961, 181.5525226013977260, -125.5803486369882478 ) ) ;
#2850=ORIENTED_EDGE ( 'NONE', *, *, #740, .F. ) ;
#2880=COLOUR_RGB ( '', 0.72549020, 0.75294118, 0.79215686) ;
#2899=AXIS2_PLACEMENT_3D ( 'NONE', #9260, #4572, #9195 ) ;
#2906=CARTESIAN_POINT ( 'NONE',  ( -19.99999999999999645, 168.0000000000000000, -124.6807709998038405 ) ) ;
#2925=ORIENTED_EDGE ( 'NONE', *, *, #616, .T. ) ;
#2932=ORIENTED_EDGE ( 'NONE', *, *, #3197, .F. ) ;
#2933=EDGE_CURVE ( 'NONE', #3651, #2975, #12075, .T. ) ;
#2942=ORIENTED_EDGE ( 'NONE', *, *, #8998, .T. ) ;
#2948=DIRECTION ( 'NONE',  ( -0.9501779778103313090, 0.000000000000000000, -0.3117078928809301486 ) ) ;
#2949=CARTESIAN_POINT ( 'NONE',  ( 20.00000000000000000, 197.0000000000000000, -124.6807709998038405 ) ) ;
#2952=FACE_OUTER_BOUND ( 'NONE', #7516, .T. ) ;
#2953=CARTESIAN_POINT ( 'NONE',  ( -19.98796572164149410, 179.0001281253265120, -125.5771477015080677 ) ) ;
#2971=CARTESIAN_POINT ( 'NONE',  ( 19.97870119493365237, 182.4301677028706479, -123.7432126472026823 ) ) ;
#2974=ORIENTED_EDGE ( 'NONE', *, *, #4663, .T. ) ;
#2975=VERTEX_POINT ( 'NONE', #4831 ) ;
#2978=CARTESIAN_POINT ( 'NONE',  ( -21.06515428438344273, 181.3786429727620089, -125.8502496116465039 ) ) ;
#2990=ORIENTED_EDGE ( 'NONE', *, *, #47, .T. ) ;
#3001=ORIENTED_EDGE ( 'NONE', *, *, #8640, .F. ) ;
#3007=B_SPLINE_CURVE_WITH_KNOTS ( 'NONE', 3,
 ( #4963, #4452, #3505, #677, #10012, #7297, #11588, #2189, #1322, #4330, #3109, #9668, #9723, #6882, #7878, #1261, #8100, #8741, #1206, #5956 ),
 .UNSPECIFIED., .F., .F.,
 ( 4, 2, 2, 2, 2, 2, 2, 2, 2, 4 ),
 ( 0.0001175641502471066547, 0.0008018704293974582287, 0.001486176708547809911, 0.002170482987698161160, 0.002854789266848512842, 0.003539095545998864525, 0.004223401825149216207, 0.004907708104299568323, 0.005249861243874702314, 0.005592014383449837173 ),
 .UNSPECIFIED. ) ;
#3008=DIRECTION ( 'NONE',  ( 0.3117078928809249860, 1.670400663243698742E-14, -0.9501779778103330854 ) ) ;
#3010=CIRCLE ( 'NONE', #6162, 1.000000000000000000 ) ;
#3050=CARTESIAN_POINT ( 'NONE',  ( 19.99672548776941383, 177.7005832697889787, -125.1535681142731420 ) ) ;
#3072=ADVANCED_FACE ( 'NONE', ( #11865 ), #12139, .T. ) ;
#3079=CARTESIAN_POINT ( 'NONE',  ( 19.91065551487656293, 178.8801318698700129, -122.7901100908945011 ) ) ;
#3080=CARTESIAN_POINT ( 'NONE',  ( -19.98803719849065885, 181.4113409838737425, -123.7644832658072289 ) ) ;
#3089=CARTESIAN_POINT ( 'NONE',  ( -20.71964524312745937, 180.2041921146310415, -123.3053720114591272 ) ) ;
#3109=CARTESIAN_POINT ( 'NONE',  ( -19.89960222275902524, 181.8553529586133379, -126.6887416412435243 ) ) ;
#3115=ORIENTED_EDGE ( 'NONE', *, *, #8190, .T. ) ;
#3122=AXIS2_PLACEMENT_3D ( 'NONE', #9247, #9183, #8138 ) ;
#3126=AXIS2_PLACEMENT_3D ( 'NONE', #2156, #8706, #8824 ) ;
#3135=CARTESIAN_POINT ( 'NONE',  ( 20.00000000000000000, 177.7280889209192480, -124.4725468461322890 ) ) ;
#3142=VECTOR ( 'NONE', #10799, 1000.000000000000000 ) ;
#3144=CARTESIAN_POINT ( 'NONE',  ( 21.06286287744583774, 178.9509521733696715, -125.7496676813577068 ) ) ;
#3145=CARTESIAN_POINT ( 'NONE',  ( 4.216865464401061553E-15, 168.0000000000000000, -124.6807709998038405 ) ) ;
#3151=B_SPLINE_CURVE_WITH_KNOTS ( 'NONE', 3,
 ( #513, #6897, #10843, #10788, #4238, #8011, #10665, #5037, #2325, #2377, #7072, #3297 ),
 .UNSPECIFIED., .F., .F.,
 ( 4, 2, 2, 2, 2, 4 ),
 ( 0.01304329750449841063, 0.01337875200764213762, 0.01371420651078590625, 0.01438511551707342788, 0.01505602452336094951, 0.01572693352964846941 ),
 .UNSPECIFIED. ) ;
#3167=CARTESIAN_POINT ( 'NONE',  ( -19.99999999999988276, 177.7282845042021791, -124.4700813638023931 ) ) ;
#3175=ORIENTED_EDGE ( 'NONE', *, *, #2837, .T. ) ;
#3197=EDGE_CURVE ( 'NONE', #505, #5440, #6157, .T. ) ;
#3202=VECTOR ( 'NONE', #9556, 1000.000000000000000 ) ;
#3211=CARTESIAN_POINT ( 'NONE',  ( 7.750278301654327006E-16, 197.0000000000000000, -124.6807709998038405 ) ) ;
#3216=EDGE_CURVE ( 'NONE', #10417, #11203, #6289, .T. ) ;
#3234=UNCERTAINTY_MEASURE_WITH_UNIT (LENGTH_MEASURE( 1.000000000000000082E-05 ), #2382, 'distance_accuracy_value', 'NONE');
#3252=CARTESIAN_POINT ( 'NONE',  ( -20.00000000000014211, 182.6816575896965844, -124.4897194826051816 ) ) ;
#3255=STYLED_ITEM ( 'NONE', ( #4685 ), #12079 ) ;
#3270=EDGE_CURVE ( 'NONE', #9028, #7054, #10825, .T. ) ;
#3291=CARTESIAN_POINT ( 'NONE',  ( -8.499999999999998224, 166.0000000000000000, -124.6807709998038405 ) ) ;
#3297=CARTESIAN_POINT ( 'NONE',  ( -19.87519864879851994, 178.8871479037923393, -126.9115732480538838 ) ) ;
#3308=CARTESIAN_POINT ( 'NONE',  ( -21.04833203300971789, 181.6140747827068935, -125.4344175246748563 ) ) ;
#3326=CARTESIAN_POINT ( 'NONE',  ( 19.96127628319862879, 179.8817259792408549, -123.2228033267029019 ) ) ;
#3332=DIRECTION ( 'NONE',  ( -1.186840563529527301E-16, 1.000000000000000000, -0.000000000000000000 ) ) ;
#3346=ORIENTED_EDGE ( 'NONE', *, *, #2837, .F. ) ;
#3349=CARTESIAN_POINT ( 'NONE',  ( -21.06729583384051097, 179.4139655881280078, -126.1965993184190040 ) ) ;
#3350=ADVANCED_FACE ( 'NONE', ( #5926 ), #7479, .T. ) ;
#3357=CARTESIAN_POINT ( 'NONE',  ( -20.71964524312745581, 180.0381522043864777, -123.3053720114591130 ) ) ;
#3363=CARTESIAN_POINT ( 'NONE',  ( 20.00000000000000000, 182.6968134406613160, -124.6807709998155076 ) ) ;
#3364=CARTESIAN_POINT ( 'NONE',  ( -20.87185099990339410, 181.4830870518408972, -123.9928801481976564 ) ) ;
#3378=ORIENTED_EDGE ( 'NONE', *, *, #1523, .F. ) ;
#3379=CARTESIAN_POINT ( 'NONE',  ( -19.89107406457440774, 179.2763954864628602, -122.5941855233586466 ) ) ;
#3392=ORIENTED_EDGE ( 'NONE', *, *, #5946, .T. ) ;
#3399=DIRECTION ( 'NONE',  ( -1.224646799147353207E-16, -1.453460497224676649E-32, 1.000000000000000000 ) ) ;
#3413=AXIS2_PLACEMENT_3D ( 'NONE', #4372, #5546, #6594 ) ;
#3442=DIRECTION ( 'NONE',  ( 1.186840563529527301E-16, -1.000000000000000000, 0.000000000000000000 ) ) ;
#3444=CARTESIAN_POINT ( 'NONE',  ( 19.99747163337677591, 182.7034818914266339, -125.0350401822433497 ) ) ;
#3447=CARTESIAN_POINT ( 'NONE',  ( 20.74743244309822288, 180.7984090500023626, -123.4190994394879937 ) ) ;
#3448=EDGE_CURVE ( 'NONE', #4344, #2975, #4904, .T. ) ;
#3460=CARTESIAN_POINT ( 'NONE',  ( -19.97716120749745627, 179.8971463893286398, -126.1313698542638235 ) ) ;
#3467=DIRECTION ( 'NONE',  ( -1.000000000000000000, -1.186840563529527301E-16, 0.000000000000000000 ) ) ;
#3478=CARTESIAN_POINT ( 'NONE',  ( -20.75374193024407887, 179.5597222894005256, -123.4475611661679864 ) ) ;
#3491=CARTESIAN_POINT ( 'NONE',  ( -20.84834133081599106, 179.0338598627802753, -123.8893051224479507 ) ) ;
#3496=CARTESIAN_POINT ( 'NONE',  ( -13.32222501832919193, 180.2041921146325762, -184.1652315311841051 ) ) ;
#3502=CARTESIAN_POINT ( 'NONE',  ( 21.06462418130824688, 181.3953932437717924, -125.8282119242440871 ) ) ;
#3505=CARTESIAN_POINT ( 'NONE',  ( -19.85143985168299352, 179.2905725846962639, -127.1146981247506744 ) ) ;
#3509=CIRCLE ( 'NONE', #5292, 8.500000000000003553 ) ;
#3522=B_SPLINE_CURVE_WITH_KNOTS ( 'NONE', 3,
 ( #1520, #10853, #4251, #7668, #3956, #2971, #2270, #6159, #6733, #3363 ),
 .UNSPECIFIED., .F., .F.,
 ( 4, 2, 2, 2, 4 ),
 ( 0.007575694888659623323, 0.008165068094779329502, 0.008754441300899034814, 0.009343814507018741861, 0.009933187713138447172 ),
 .UNSPECIFIED. ) ;
#3524=CARTESIAN_POINT ( 'NONE',  ( -19.84415231186486395, 179.4841820921725173, -127.1732901015634951 ) ) ;
#3530=DIRECTION ( 'NONE',  ( 0.3117078928809249860, -1.670400663243698742E-14, 0.9501779778103330854 ) ) ;
#3532=CARTESIAN_POINT ( 'NONE',  ( 19.88188653267749118, 178.7826062614507805, -126.8526954990893927 ) ) ;
#3541=CYLINDRICAL_SURFACE ( 'NONE', #9805, 20.00000000000000000 ) ;
#3544=CARTESIAN_POINT ( 'NONE',  ( 19.97657674272267769, 180.1017299760444530, -126.1590557403436037 ) ) ;
#3548=CARTESIAN_POINT ( 'NONE',  ( -19.97250828649639587, 179.3956025841652888, -123.4200681550201892 ) ) ;
#3560=CARTESIAN_POINT ( 'NONE',  ( 19.99933548561055829, 181.6672375346512922, -124.2941161999968926 ) ) ;
#3562=ORIENTED_EDGE ( 'NONE', *, *, #12191, .F. ) ;
#3575=ORIENTED_EDGE ( 'NONE', *, *, #3988, .T. ) ;
#3577=CARTESIAN_POINT ( 'NONE',  ( -20.75789059648688095, 180.8764387032748004, -123.4649828651695458 ) ) ;
#3578=ORIENTED_EDGE ( 'NONE', *, *, #2552, .T. ) ;
#3582=CARTESIAN_POINT ( 'NONE',  ( -21.06729583384051097, 179.4139655881280078, -126.1965993184190040 ) ) ;
#3583=CARTESIAN_POINT ( 'NONE',  ( -27.10787553788293280, 180.2041921146317236, -137.3302880892917983 ) ) ;
#3596=FACE_OUTER_BOUND ( 'NONE', #10705, .T. ) ;
#3605=ORIENTED_EDGE ( 'NONE', *, *, #12191, .T. ) ;
#3613=CARTESIAN_POINT ( 'NONE',  ( -19.93794579528156419, 178.4740307436693740, -123.1021291661558195 ) ) ;
#3624=CARTESIAN_POINT ( 'NONE',  ( 21.06618838917721348, 180.8542587794627821, -126.2858731283988618 ) ) ;
#3630=CARTESIAN_POINT ( 'NONE',  ( 20.91924760697977703, 181.5974164329501264, -124.2866227082428736 ) ) ;
#3650=CARTESIAN_POINT ( 'NONE',  ( 19.86004308345772529, 179.1220966913736277, -127.0453612081607844 ) ) ;
#3651=VERTEX_POINT ( 'NONE', #2181 ) ;
#3660=DIRECTION ( 'NONE',  ( -1.186840563529527301E-16, 1.000000000000000000, -0.000000000000000000 ) ) ;
#3662=( GEOMETRIC_REPRESENTATION_CONTEXT ( 3 ) GLOBAL_UNCERTAINTY_ASSIGNED_CONTEXT ( ( #3234 ) ) GLOBAL_UNIT_ASSIGNED_CONTEXT ( ( #2382, #6221, #588 ) ) REPRESENTATION_CONTEXT ( 'NONE', 'WORKASPACE' ) );
#3669=CARTESIAN_POINT ( 'NONE',  ( 19.98760292801598126, 179.0152138695270594, -125.5961219049576982 ) ) ;
#3672=CARTESIAN_POINT ( 'NONE',  ( 1.734723475976807094E-15, 180.2041921146324910, -179.7948474705909234 ) ) ;
#3683=CARTESIAN_POINT ( 'NONE',  ( 20.71964524312746647, 180.2041921146487766, -123.3053720114591414 ) ) ;
#3689=CARTESIAN_POINT ( 'NONE',  ( -20.76475501013377212, 179.4826916305587474, -123.4955357876650197 ) ) ;
#3695=ORIENTED_EDGE ( 'NONE', *, *, #2552, .F. ) ;
#3698=CARTESIAN_POINT ( 'NONE',  ( 20.79565762252865468, 181.1410762094974700, -123.6324090417393649 ) ) ;
#3722=CARTESIAN_POINT ( 'NONE',  ( -19.96948860049111474, 182.3247467770471530, -123.5689856398053763 ) ) ;
#3726=EDGE_CURVE ( 'NONE', #154, #6278, #1172, .T. ) ;
#3761=CARTESIAN_POINT ( 'NONE',  ( 21.04760817881890844, 181.6185052388174199, -125.4224630414783945 ) ) ;
#3767=CARTESIAN_POINT ( 'NONE',  ( 21.06714545844871367, 179.4370239411119030, -126.2109676220344596 ) ) ;
#3791=CARTESIAN_POINT ( 'NONE',  ( 21.06714545844871722, 179.4370239411119030, -126.2109676220344596 ) ) ;
#3800=SURFACE_SIDE_STYLE ('',( #11407 ) ) ;
#3810=CARTESIAN_POINT ( 'NONE',  ( -19.99208445718651106, 177.7326588799362810, -125.2637803837037325 ) ) ;
#3814=TOROIDAL_SURFACE ( 'NONE', #10723, 14.02076803445813269, 1.499999999999998002 ) ;
#3819=CARTESIAN_POINT ( 'NONE',  ( 19.90005091283025962, 178.5478491056598500, -126.6842376513516513 ) ) ;
#3824=EDGE_LOOP ( 'NONE', ( #1784, #9547, #6141, #9948, #712, #7860 ) ) ;
#3829=CARTESIAN_POINT ( 'NONE',  ( 11.89695805161205655, 180.2041921146325762, -183.6976696918629557 ) ) ;
#3831=DIRECTION ( 'NONE',  ( -1.186840563529527301E-16, 1.000000000000000000, -0.000000000000000000 ) ) ;
#3833=ORIENTED_EDGE ( 'NONE', *, *, #5265, .T. ) ;
#3841=CARTESIAN_POINT ( 'NONE',  ( 20.80735028308761869, 179.2184937932714490, -123.6883961446522022 ) ) ;
#3842=AXIS2_PLACEMENT_3D ( 'NONE', #7204, #9111, #2499 ) ;
#3843=CARTESIAN_POINT ( 'NONE',  ( -19.99390413358784357, 181.6003807074973793, -125.2540357159168423 ) ) ;
#3854=CIRCLE ( 'NONE', #10167, 0.9999999999999991118 ) ;
#3856=CARTESIAN_POINT ( 'NONE',  ( 19.99326885945900401, 178.8248732837839157, -125.2918954700392646 ) ) ;
#3870=CARTESIAN_POINT ( 'NONE',  ( -18.99999999999999645, 167.0000000000000000, -124.6807709998038405 ) ) ;
#3874=CARTESIAN_POINT ( 'NONE',  ( -19.95650872578057644, 177.9942513821760031, -126.0067755081681042 ) ) ;
#3884=CARTESIAN_POINT ( 'NONE',  ( 20.00000000000000711, 177.6938224469233774, -124.9045029178196842 ) ) ;
#3885=EDGE_CURVE ( 'NONE', #2975, #3899, #791, .T. ) ;
#3886=CARTESIAN_POINT ( 'NONE',  ( -20.79945932778137063, 181.1616795883780071, -123.6498693937513025 ) ) ;
#3899=VERTEX_POINT ( 'NONE', #3829 ) ;
#3900=EDGE_LOOP ( 'NONE', ( #10586, #2403, #5949, #10431 ) ) ;
#3901=CARTESIAN_POINT ( 'NONE',  ( 19.96555171194421163, 178.1301448319365193, -123.4995670770394582 ) ) ;
#3903=CARTESIAN_POINT ( 'NONE',  ( -19.97681936893992116, 182.4076374096303539, -123.7075806145273873 ) ) ;
#3935=AXIS2_PLACEMENT_3D ( 'NONE', #292, #1059, #4818 ) ;
#3937=DIRECTION ( 'NONE',  ( -0.000000000000000000, -1.000000000000000000, -1.757987137413040192E-14 ) ) ;
#3947=ORIENTED_EDGE ( 'NONE', *, *, #4181, .T. ) ;
#3955=DIRECTION ( 'NONE',  ( -1.000000000000000000, 0.000000000000000000, 0.000000000000000000 ) ) ;
#3956=CARTESIAN_POINT ( 'NONE',  ( 19.96040119434836768, 182.2179960502109850, -123.4119521547231386 ) ) ;
#3988=EDGE_CURVE ( 'NONE', #2611, #3899, #9271, .T. ) ;
#3994=CYLINDRICAL_SURFACE ( 'NONE', #11547, 1.500000000000000444 ) ;
#3998=CARTESIAN_POINT ( 'NONE',  ( -19.92650117820961952, 178.2666534087950367, -126.3986386542856337 ) ) ;
#4007=DIRECTION ( 'NONE',  ( -1.000000000000000000, 0.000000000000000000, 0.000000000000000000 ) ) ;
#4011=EDGE_LOOP ( 'NONE', ( #2850, #4469, #11180, #7431 ) ) ;
#4019=VERTEX_POINT ( 'NONE', #295 ) ;
#4027=ORIENTED_EDGE ( 'NONE', *, *, #8998, .F. ) ;
#4031=DIRECTION ( 'NONE',  ( 1.186840563529527301E-16, -1.000000000000000000, 0.000000000000000000 ) ) ;
#4036=DIRECTION ( 'NONE',  ( 0.9501779778103313090, 0.000000000000000000, -0.3117078928809301486 ) ) ;
#4037=EDGE_CURVE ( 'NONE', #7759, #505, #574, .T. ) ;
#4042=AXIS2_PLACEMENT_3D ( 'NONE', #12005, #8970, #8904 ) ;
#4046=CARTESIAN_POINT ( 'NONE',  ( 19.99813415626286783, 177.7525720880900053, -124.3666714923229222 ) ) ;
#4051=DIRECTION ( 'NONE',  ( 1.000000000000000000, 1.186840563529527301E-16, 0.000000000000000000 ) ) ;
#4055=AXIS2_PLACEMENT_3D ( 'NONE', #556, #618, #2474 ) ;
#4065=CARTESIAN_POINT ( 'NONE',  ( -19.98030737385957423, 179.4757119253121402, -125.9751133749524712 ) ) ;
#4074=CARTESIAN_POINT ( 'NONE',  ( 19.95569904651928184, 178.2465785626148431, -123.3391210327002199 ) ) ;
#4079=CARTESIAN_POINT ( 'NONE',  ( 1.734723475976807094E-15, 180.2041921146324910, -179.7948474705909234 ) ) ;
#4089=FACE_OUTER_BOUND ( 'NONE', #5677, .T. ) ;
#4097=CARTESIAN_POINT ( 'NONE',  ( -29.03136272649514638, 180.2041921146316668, -134.6807709998038547 ) ) ;
#4106=CARTESIAN_POINT ( 'NONE',  ( -19.87821795393918478, 180.7372106301276062, -122.4761893939201940 ) ) ;
#4130=CARTESIAN_POINT ( 'NONE',  ( 19.98454104437637824, 177.9140520261175311, -123.8699308089654778 ) ) ;
#4132=EDGE_LOOP ( 'NONE', ( #2816, #9607 ) ) ;
#4139=CIRCLE ( 'NONE', #983, 1.499999999999998224 ) ;
#4152=CARTESIAN_POINT ( 'NONE',  ( 20.00000000000000000, 196.0000000000000000, -124.6807709998038405 ) ) ;
#4158=( BOUNDED_SURFACE ( )  B_SPLINE_SURFACE ( 3, 2, ( 
 ( #10886, #8969, #3582 ),
 ( #5259, #9027, #7372 ),
 ( #567, #2670, #6444 ),
 ( #3524, #4348, #10087 ),
 ( #11146, #3460, #7315 ),
 ( #4538, #1620, #6378 ),
 ( #2545, #8115, #10954 ),
 ( #9090, #497, #2417 ),
 ( #5443, #4402, #2483 ),
 ( #11880, #6259, #10028 ),
 ( #11943, #1555, #630 ),
 ( #6318, #5377, #9221 ),
 ( #8314, #9156, #4470 ),
 ( #12074, #9290, #2978 ),
 ( #1934, #2799, #11384 ),
 ( #4722, #4603, #4665 ),
 ( #11212, #5697, #2737 ),
 ( #9469, #3843, #4829 ),
 ( #6504, #1814, #8443 ),
 ( #9528, #11447, #127 ),
 ( #1009, #894, #7618 ),
 ( #830, #1995, #5578 ),
 ( #8374, #6568, #10460 ),
 ( #3903, #9351, #12202 ),
 ( #3722, #7676, #1876 ),
 ( #8497, #3080, #162 ),
 ( #1912, #4755, #3886 ),
 ( #5676, #11378, #44 ) ),
 .UNSPECIFIED., .F., .F., .F. ) 
 B_SPLINE_SURFACE_WITH_KNOTS ( ( 4, 2, 2, 2, 2, 2, 2, 2, 2, 2, 2, 2, 2, 4 ),
 ( 3, 3 ),
 ( 0.000000000000000000, 0.0004930383923902153772, 0.0009860767847804307543, 0.001479115177170646240, 0.001972153569560861509, 0.002958230354341292480, 0.003451268746731507749, 0.003944307139121723017, 0.004437345531511939153, 0.004930383923902154422, 0.005916460708682584960, 0.006409499101072800228, 0.006902537493463015497, 0.007888614278243446035 ),
 ( 0.000000000000000000, 1.000000000000000000 ),
 .UNSPECIFIED. ) 
 GEOMETRIC_REPRESENTATION_ITEM ( )  RATIONAL_B_SPLINE_SURFACE ( (
 ( 1.000000000000000000, 0.6689879873414465994, 1.000000000000000000),
 ( 1.000000000000000000, 0.6682619615833934601, 1.000000000000000000),
 ( 1.000000000000000000, 0.6677734440439352381, 1.000000000000000000),
 ( 1.000000000000000000, 0.6670763045104984856, 1.000000000000000000),
 ( 1.000000000000000000, 0.6668655740656856956, 1.000000000000000000),
 ( 1.000000000000000000, 0.6666182310250359233, 1.000000000000000000),
 ( 1.000000000000000000, 0.6665784742421086984, 1.000000000000000000),
 ( 1.000000000000000000, 0.6666353228050939661, 1.000000000000000000),
 ( 1.000000000000000000, 0.6667346642862397310, 1.000000000000000000),
 ( 1.000000000000000000, 0.6673328464405002824, 1.000000000000000000),
 ( 1.000000000000000000, 0.6681342971656755170, 1.000000000000000000),
 ( 1.000000000000000000, 0.6708694338352457764, 1.000000000000000000),
 ( 1.000000000000000000, 0.6720569605147309611, 1.000000000000000000),
 ( 1.000000000000000000, 0.6751225054005377535, 1.000000000000000000),
 ( 1.000000000000000000, 0.6769812796920648967, 1.000000000000000000),
 ( 1.000000000000000000, 0.6815111439571803764, 1.000000000000000000),
 ( 1.000000000000000000, 0.6842124604620484218, 1.000000000000000000),
 ( 1.000000000000000000, 0.6903314890518940095, 1.000000000000000000),
 ( 1.000000000000000000, 0.6937642806658218531, 1.000000000000000000),
 ( 1.000000000000000000, 0.7052556801245680740, 1.000000000000000000),
 ( 1.000000000000000000, 0.7142546037275387949, 1.000000000000000000),
 ( 1.000000000000000000, 0.7287603549096577371, 1.000000000000000000),
 ( 1.000000000000000000, 0.7336520540315742966, 1.000000000000000000),
 ( 1.000000000000000000, 0.7434275992171806013, 1.000000000000000000),
 ( 1.000000000000000000, 0.7483638594814020495, 1.000000000000000000),
 ( 1.000000000000000000, 0.7624769318894530912, 1.000000000000000000),
 ( 1.000000000000000000, 0.7710581372201869010, 1.000000000000000000),
 ( 1.000000000000000000, 0.7778924984312529656, 1.000000000000000000) ) ) 
 REPRESENTATION_ITEM ( '' )  SURFACE ( )  );
#4171=CARTESIAN_POINT ( 'NONE',  ( -21.06240745282767080, 180.2041921146517041, -126.4269926335259413 ) ) ;
#4181=EDGE_CURVE ( 'NONE', #4517, #6610, #3522, .T. ) ;
#4182=CARTESIAN_POINT ( 'NONE',  ( -28.53314250459843038, 180.2041921146317236, -137.7978499286131751 ) ) ;
#4185=CARTESIAN_POINT ( 'NONE',  ( 19.88975813659335756, 181.1020309933168164, -122.5829583614533362 ) ) ;
#4189=LINE ( 'NONE', #465, #3142 ) ;
#4190=CARTESIAN_POINT ( 'NONE',  ( -19.99715534307563658, 182.6423572728569980, -124.2973801271140246 ) ) ;
#4202=EDGE_CURVE ( 'NONE', #1329, #822, #6877, .T. ) ;
#4205=CARTESIAN_POINT ( 'NONE',  ( 19.87222254682778910, 180.2228354577052301, -122.4235914049322389 ) ) ;
#4206=ADVANCED_FACE ( 'NONE', ( #11789 ), #7023, .T. ) ;
#4208=CARTESIAN_POINT ( 'NONE',  ( 2.510525938252074008E-14, -7.999999999999979572, -124.6807709998038405 ) ) ;
#4225=CARTESIAN_POINT ( 'NONE',  ( 8.500000000000008882, 166.0000000000000000, -124.6807709998038405 ) ) ;
#4226=ORIENTED_EDGE ( 'NONE', *, *, #3270, .T. ) ;
#4229=AXIS2_PLACEMENT_3D ( 'NONE', #4097, #9018, #7927 ) ;
#4235=APPLICATION_CONTEXT ( 'automotive_design' ) ;
#4238=CARTESIAN_POINT ( 'NONE',  ( -19.99263453218006603, 177.7304828429992654, -125.2341356145629732 ) ) ;
#4245=CARTESIAN_POINT ( 'NONE',  ( 11.89695805161204234, 180.2041921146325762, -183.6976696918630125 ) ) ;
#4250=B_SPLINE_CURVE_WITH_KNOTS ( 'NONE', 3,
 ( #8584, #9327, #3819, #1731, #1054, #108, #9509, #6604, #3884, #8350 ),
 .UNSPECIFIED., .F., .F.,
 ( 4, 2, 2, 2, 4 ),
 ( 0.01531771418541752645, 0.01599364935748912725, 0.01666958452956072631, 0.01734551970163232884, 0.01802145487370392790 ),
 .UNSPECIFIED. ) ;
#4251=CARTESIAN_POINT ( 'NONE',  ( 19.92885329534479055, 181.8094058714599157, -122.9898942296876356 ) ) ;
#4252=CARTESIAN_POINT ( 'NONE',  ( -20.94548197283593893, 181.6568612240360210, -124.4525847695740310 ) ) ;
#4254=CARTESIAN_POINT ( 'NONE',  ( 19.97670222400810758, 180.3732814399037068, -126.1531159571454310 ) ) ;
#4256=CARTESIAN_POINT ( 'NONE',  ( 19.87445315872311369, 179.8633251070327219, -122.4428743481628601 ) ) ;
#4286=EDGE_LOOP ( 'NONE', ( #980, #9292, #2974, #3947, #2990, #7688, #4027, #6578, #9280, #3378 ) ) ;
#4300=FACE_OUTER_BOUND ( 'NONE', #7491, .T. ) ;
#4310=DIRECTION ( 'NONE',  ( 1.186840563529527301E-16, -1.000000000000000000, 0.000000000000000000 ) ) ;
#4318=EDGE_LOOP ( 'NONE', ( #11882, #6547, #5750, #2932, #1803, #289 ) ) ;
#4323=DIRECTION ( 'NONE',  ( -1.186840563529527301E-16, 1.000000000000000000, -0.000000000000000000 ) ) ;
#4330=CARTESIAN_POINT ( 'NONE',  ( -19.88499600238774434, 181.6747900880826592, -126.8253906927961623 ) ) ;
#4342=EDGE_CURVE ( 'NONE', #6027, #10270, #8850, .T. ) ;
#4344=VERTEX_POINT ( 'NONE', #5281 ) ;
#4346=EDGE_CURVE ( 'NONE', #2139, #4019, #7474, .T. ) ;
#4348=CARTESIAN_POINT ( 'NONE',  ( -19.97760348394007579, 179.8079052437743997, -126.1102380945337558 ) ) ;
#4351=CARTESIAN_POINT ( 'NONE',  ( 2.498657532616778856E-14, -6.999999999999978684, -124.6807709998038405 ) ) ;
#4360=DIRECTION ( 'NONE',  ( 1.000000000000000000, 0.000000000000000000, 0.000000000000000000 ) ) ;
#4364=CARTESIAN_POINT ( 'NONE',  ( -20.72699427085588297, 179.8710689655571855, -123.3349751025961325 ) ) ;
#4372=CARTESIAN_POINT ( 'NONE',  ( 20.90408460058374729, 181.4799304009739842, -122.6759650212516561 ) ) ;
#4379=CYLINDRICAL_SURFACE ( 'NONE', #839, 7.500000000000005329 ) ;
#4382=AXIS2_PLACEMENT_3D ( 'NONE', #5129, #303, #5237 ) ;
#4383=CARTESIAN_POINT ( 'NONE',  ( 19.92456121491558463, 181.7656274153872573, -122.9373171337986008 ) ) ;
#4386=CARTESIAN_POINT ( 'NONE',  ( 19.90865200055594997, 181.4799304009739842, -122.7714319726112819 ) ) ;
#4388=CARTESIAN_POINT ( 'NONE',  ( 8.937118865183856033E-16, 196.0000000000000000, -124.6807709998038405 ) ) ;
#4398=AXIS2_PLACEMENT_3D ( 'NONE', #5701, #7558, #4036 ) ;
#4402=CARTESIAN_POINT ( 'NONE',  ( -19.97689317482322480, 180.4398926601855067, -126.1441920888607058 ) ) ;
#4415=CARTESIAN_POINT ( 'NONE',  ( 20.94276857858305618, 181.6519786105751848, -124.4341959704801610 ) ) ;
#4427=DIRECTION ( 'NONE',  ( 0.000000000000000000, -0.000000000000000000, -1.000000000000000000 ) ) ;
#4431=DIRECTION ( 'NONE',  ( -1.000000000000000000, 0.000000000000000000, 0.000000000000000000 ) ) ;
#4435=CARTESIAN_POINT ( 'NONE',  ( -19.87230422438681288, 180.2683866676943296, -122.4243209296576680 ) ) ;
#4449=CARTESIAN_POINT ( 'NONE',  ( 21.01102415922771982, 181.7037659814379538, -124.9847730909611130 ) ) ;
#4452=CARTESIAN_POINT ( 'NONE',  ( -19.86218813316839160, 179.0832429894416862, -127.0274896556490631 ) ) ;
#4467=CARTESIAN_POINT ( 'NONE',  ( -20.71964524312745937, 180.2041921146310415, -123.3053720114591272 ) ) ;
#4469=ORIENTED_EDGE ( 'NONE', *, *, #9412, .F. ) ;
#4470=CARTESIAN_POINT ( 'NONE',  ( -21.06761139726929244, 181.2453226294160515, -126.0007492840280179 ) ) ;
#4473=DIRECTION ( 'NONE',  ( 1.000000000000000000, 0.000000000000000000, 0.000000000000000000 ) ) ;
#4474=VERTEX_POINT ( 'NONE', #12167 ) ;
#4491=ORIENTED_EDGE ( 'NONE', *, *, #6929, .T. ) ;
#4499=CARTESIAN_POINT ( 'NONE',  ( -19.96087997506392142, 179.9125189710396739, -123.2164587046221271 ) ) ;
#4513=CARTESIAN_POINT ( 'NONE',  ( 19.99920057787401717, 181.7064984983803129, -124.8736205325594284 ) ) ;
#4517=VERTEX_POINT ( 'NONE', #5601 ) ;
#4527=CARTESIAN_POINT ( 'NONE',  ( 20.77152989773913916, 180.9696350864299461, -123.5256872951201643 ) ) ;
#4535=CARTESIAN_POINT ( 'NONE',  ( 19.87268743161337170, 178.9255784920988503, -126.9338343023757290 ) ) ;
#4538=CARTESIAN_POINT ( 'NONE',  ( -19.83253561012729449, 179.9725903414323795, -127.2636293852243483 ) ) ;
#4540=ORIENTED_EDGE ( 'NONE', *, *, #5688, .F. ) ;
#4547=CARTESIAN_POINT ( 'NONE',  ( 21.06147608529250803, 178.9413095352420271, -125.7232933582278491 ) ) ;
#4555=SURFACE_STYLE_USAGE ( .BOTH. , #3800 ) ;
#4563=CARTESIAN_POINT ( 'NONE',  ( -19.95977122504825729, 180.0239105065436434, -123.1990849849620844 ) ) ;
#4564=DIRECTION ( 'NONE',  ( -1.000000000000000000, -1.186840563529527301E-16, 0.000000000000000000 ) ) ;
#4572=DIRECTION ( 'NONE',  ( -1.186840563529527301E-16, 1.000000000000000000, 0.000000000000000000 ) ) ;
#4580=CARTESIAN_POINT ( 'NONE',  ( 19.97971902011833123, 180.8960314115462040, -126.0058985864737053 ) ) ;
#4590=ORIENTED_EDGE ( 'NONE', *, *, #3885, .F. ) ;
#4597=CARTESIAN_POINT ( 'NONE',  ( 19.97025581332069422, 182.5233676713443174, -125.7761851878406105 ) ) ;
#4603=CARTESIAN_POINT ( 'NONE',  ( -19.98958826779223230, 181.4702305597406848, -125.4918071840122735 ) ) ;
#4625=CARTESIAN_POINT ( 'NONE',  ( -6.499999999999979572, -6.999999999999979572, -124.6807709998038405 ) ) ;
#4630=CARTESIAN_POINT ( 'NONE',  ( -19.87341384624713569, 180.4358019248037692, -122.4339773266618323 ) ) ;
#4631=CARTESIAN_POINT ( 'NONE',  ( 14.74749198504306591, 180.2041921146325762, -184.6327933705057376 ) ) ;
#4632=CIRCLE ( 'NONE', #10729, 1.499999999999999112 ) ;
#4644=CARTESIAN_POINT ( 'NONE',  ( 19.99652087076804818, 181.6001326330613779, -124.1032781992507523 ) ) ;
#4663=EDGE_CURVE ( 'NONE', #6035, #4517, #9888, .T. ) ;
#4665=CARTESIAN_POINT ( 'NONE',  ( -21.05626678059735823, 181.5387050158279010, -125.5955412462414813 ) ) ;
#4679=AXIS2_PLACEMENT_3D ( 'NONE', #3496, #11051, #8806 ) ;
#4685=PRESENTATION_STYLE_ASSIGNMENT (( #4555 ) ) ;
#4686=ORIENTED_EDGE ( 'NONE', *, *, #307, .F. ) ;
#4690=CARTESIAN_POINT ( 'NONE',  ( 20.77152989773913916, 180.9696350864299461, -123.5256872951201643 ) ) ;
#4696=CARTESIAN_POINT ( 'NONE',  ( -20.99418893176411416, 178.7017074851977156, -124.8287954103437301 ) ) ;
#4705=DIRECTION ( 'NONE',  ( -0.3117078928809153826, -1.979053562451413181E-14, -0.9501779778103363050 ) ) ;
#4709=DIRECTION ( 'NONE',  ( 0.000000000000000000, 1.773410419504194611E-14, -1.000000000000000000 ) ) ;
#4716=CARTESIAN_POINT ( 'NONE',  ( 19.85038338882363718, 181.0937693555581802, -127.1232350078937969 ) ) ;
#4722=CARTESIAN_POINT ( 'NONE',  ( -19.95815963485732425, 182.4283802827153806, -125.9807797667228897 ) ) ;
#4727=EDGE_CURVE ( 'NONE', #3651, #4474, #11287, .T. ) ;
#4755=CARTESIAN_POINT ( 'NONE',  ( -19.98141544511310386, 181.2666267236099884, -123.6015590193429858 ) ) ;
#4765=DIRECTION ( 'NONE',  ( 0.000000000000000000, 0.000000000000000000, -1.000000000000000000 ) ) ;
#4775=CARTESIAN_POINT ( 'NONE',  ( 20.82193910853440855, 179.1472446959528213, -123.7577175453547085 ) ) ;
#4818=DIRECTION ( 'NONE',  ( 0.9501779778103254248, 0.000000000000000000, 0.3117078928809486338 ) ) ;
#4829=CARTESIAN_POINT ( 'NONE',  ( -21.03937020940231051, 181.6480601768998895, -125.3115690614735911 ) ) ;
#4831=CARTESIAN_POINT ( 'NONE',  ( -11.89695805161369080, 180.2041921146325478, -183.6976696918626999 ) ) ;
#4841=CARTESIAN_POINT ( 'NONE',  ( 19.97899957837033824, 177.8194711809319415, -125.6095969703938096 ) ) ;
#4896=CARTESIAN_POINT ( 'NONE',  ( 4.216865464401061553E-15, 168.0000000000000000, -124.6807709998038405 ) ) ;
#4904=CIRCLE ( 'NONE', #3935, 1.500000000000000666 ) ;
#4913=CARTESIAN_POINT ( 'NONE',  ( -28.53314250459843038, 180.2041921146317236, -137.7978499286131751 ) ) ;
#4918=CARTESIAN_POINT ( 'NONE',  ( -21.04069087917613956, 178.7655007512674104, -125.3296589603482261 ) ) ;
#4928=ADVANCED_FACE ( 'NONE', ( #9704 ), #1824, .T. ) ;
#4956=ORIENTED_EDGE ( 'NONE', *, *, #5915, .T. ) ;
#4963=CARTESIAN_POINT ( 'NONE',  ( -19.87519864879851994, 178.8871479037923393, -126.9115732480538838 ) ) ;
#5017=CIRCLE ( 'NONE', #11933, 20.00000000000000000 ) ;
#5021=CARTESIAN_POINT ( 'NONE',  ( -19.90044468808352462, 181.3371914423172768, -122.6846776996206358 ) ) ;
#5034=EDGE_CURVE ( 'NONE', #154, #3651, #11088, .T. ) ;
#5037=CARTESIAN_POINT ( 'NONE',  ( -19.94620750243457863, 178.0808788782996146, -126.1595479531101631 ) ) ;
#5079=ADVANCED_FACE ( 'NONE', ( #539 ), #4379, .T. ) ;
#5107=DIRECTION ( 'NONE',  ( -0.9501779778103313090, 0.000000000000000000, -0.3117078928809301486 ) ) ;
#5113=VECTOR ( 'NONE', #2719, 1000.000000000000000 ) ;
#5129=CARTESIAN_POINT ( 'NONE',  ( 2.498657532616778856E-14, -6.999999999999978684, -124.6807709998038405 ) ) ;
#5134=DIRECTION ( 'NONE',  ( -1.000000000000000000, 0.000000000000000000, 0.000000000000000000 ) ) ;
#5141=CARTESIAN_POINT ( 'NONE',  ( 19.97976963877082923, 177.9666655783959186, -123.7712089892055189 ) ) ;
#5147=TOROIDAL_SURFACE ( 'NONE', #8121, 10.00000000000003730, 1.499999999999998002 ) ;
#5168=CIRCLE ( 'NONE', #4382, 7.500000000000005329 ) ;
#5171=CARTESIAN_POINT ( 'NONE',  ( -19.93086114385802077, 181.8378500852114712, -123.0137796683760456 ) ) ;
#5178=CIRCLE ( 'NONE', #11301, 1.000000000000000888 ) ;
#5204=CARTESIAN_POINT ( 'NONE',  ( -21.06521297978533980, 179.6586675211645741, -126.3290294770899891 ) ) ;
#5211=DIRECTION ( 'NONE',  ( -1.000000000000000000, -1.186840563529527301E-16, 0.000000000000000000 ) ) ;
#5222=CARTESIAN_POINT ( 'NONE',  ( 21.06320946107762282, 180.4881934621326991, -126.4026505290603808 ) ) ;
#5225=AXIS2_PLACEMENT_3D ( 'NONE', #520, #10972, #8133 ) ;
#5237=DIRECTION ( 'NONE',  ( -1.000000000000000000, -1.156482317317870492E-16, 0.000000000000000000 ) ) ;
#5240=CARTESIAN_POINT ( 'NONE',  ( 19.95910083177870220, 180.2168005683687113, -123.1884788074740271 ) ) ;
#5247=EDGE_CURVE ( 'NONE', #5440, #11672, #10908, .T. ) ;
#5259=CARTESIAN_POINT ( 'NONE',  ( -19.86581666024647319, 179.0285536720372477, -126.9951615115761143 ) ) ;
#5265=EDGE_CURVE ( 'NONE', #6610, #5632, #598, .T. ) ;
#5266=CARTESIAN_POINT ( 'NONE',  ( -21.06656016739612269, 179.5324992879768899, -126.2719758226758273 ) ) ;
#5275=AXIS2_PLACEMENT_3D ( 'NONE', #2580, #3442, #10930 ) ;
#5281=CARTESIAN_POINT ( 'NONE',  ( -14.74749198504467174, 180.2041921146325478, -184.6327933705055386 ) ) ;
#5282=CARTESIAN_POINT ( 'NONE',  ( -21.06240745282767080, 180.2041921146517041, -126.4269926335259413 ) ) ;
#5290=ORIENTED_EDGE ( 'NONE', *, *, #11375, .F. ) ;
#5292=AXIS2_PLACEMENT_3D ( 'NONE', #9626, #159, #221 ) ;
#5296=EDGE_CURVE ( 'NONE', #2780, #8550, #7526, .T. ) ;
#5302=ORIENTED_EDGE ( 'NONE', *, *, #1692, .F. ) ;
#5303=CARTESIAN_POINT ( 'NONE',  ( -19.99667327426407937, 177.7725865070964062, -124.2645694134507153 ) ) ;
#5313=AXIS2_PLACEMENT_3D ( 'NONE', #11291, #5779, #9618 ) ;
#5321=DIRECTION ( 'NONE',  ( 0.000000000000000000, 1.689469820081758265E-14, -1.000000000000000000 ) ) ;
#5331=CARTESIAN_POINT ( 'NONE',  ( 19.00000000000000355, 167.0000000000000000, -124.6807709998038405 ) ) ;
#5358=CARTESIAN_POINT ( 'NONE',  ( 19.97493946039394430, 182.3862959170359659, -123.6698968802414953 ) ) ;
#5360=CARTESIAN_POINT ( 'NONE',  ( -19.95507986285562652, 178.2540685118973443, -123.3298867597350323 ) ) ;
#5375=CARTESIAN_POINT ( 'NONE',  ( 19.83195864043130641, 180.4357261996970010, -127.2679348835839335 ) ) ;
#5377=CARTESIAN_POINT ( 'NONE',  ( -19.98227708713212181, 181.0992491550492787, -125.8737299293410530 ) ) ;
#5396=CIRCLE ( 'NONE', #4042, 19.00000000000000000 ) ;
#5402=EDGE_CURVE ( 'NONE', #4019, #9416, #5168, .T. ) ;
#5404=CARTESIAN_POINT ( 'NONE',  ( 20.74227355824053021, 180.7311119294840580, -123.3990510803982943 ) ) ;
#5409=CARTESIAN_POINT ( 'NONE',  ( -19.92916319319399676, 178.5949286292980389, -122.9963005650378420 ) ) ;
#5411=ORIENTED_EDGE ( 'NONE', *, *, #2933, .F. ) ;
#5421=CARTESIAN_POINT ( 'NONE',  ( 20.00026463111520414, 182.6897424871681324, -124.5631314607046818 ) ) ;
#5425=CIRCLE ( 'NONE', #914, 1.000000000000000888 ) ;
#5439=CARTESIAN_POINT ( 'NONE',  ( 19.93046079246938618, 182.1848923560334015, -126.3549534181600791 ) ) ;
#5440=VERTEX_POINT ( 'NONE', #11750 ) ;
#5443=CARTESIAN_POINT ( 'NONE',  ( -19.83578844811568587, 180.6327930221633835, -127.2386752689097023 ) ) ;
#5453=CARTESIAN_POINT ( 'NONE',  ( -19.00000000000000000, 197.0000000000000000, -124.6807709998038405 ) ) ;
#5460=CARTESIAN_POINT ( 'NONE',  ( -21.06729583384051097, 179.4139655881280078, -126.1965993184190040 ) ) ;
#5468=FACE_OUTER_BOUND ( 'NONE', #4286, .T. ) ;
#5473=CARTESIAN_POINT ( 'NONE',  ( 21.06714545844871722, 179.4370239411119030, -126.2109676220344596 ) ) ;
#5485=ORIENTED_EDGE ( 'NONE', *, *, #6929, .F. ) ;
#5486=PLANE ( 'NONE',  #2899 ) ;
#5493=CARTESIAN_POINT ( 'NONE',  ( 21.05011458093100529, 181.5921831639467996, -125.4765988369088916 ) ) ;
#5523=CARTESIAN_POINT ( 'NONE',  ( -19.91081574664456610, 181.5182364730087272, -122.7941294590837913 ) ) ;
#5535=ORIENTED_EDGE ( 'NONE', *, *, #5296, .T. ) ;
#5538=ADVANCED_FACE ( 'NONE', ( #4089 ), #6164, .T. ) ;
#5541=CARTESIAN_POINT ( 'NONE',  ( 19.87268743161337170, 178.9255784920988503, -126.9338343023757290 ) ) ;
#5545=CARTESIAN_POINT ( 'NONE',  ( -20.00054430879287892, 177.7104753434648785, -124.6347125233424009 ) ) ;
#5546=DIRECTION ( 'NONE',  ( -0.04986130261928722884, -0.8527687809245380057, 0.5199031224964757447 ) ) ;
#5556=CARTESIAN_POINT ( 'NONE',  ( 19.85181743999062576, 181.1549164222419961, -127.1121716299344087 ) ) ;
#5576=ADVANCED_FACE ( 'NONE', ( #10007 ), #7886, .F. ) ;
#5578=CARTESIAN_POINT ( 'NONE',  ( -20.93827155636993353, 181.6390200720728387, -124.4080817122161307 ) ) ;
#5587=CARTESIAN_POINT ( 'NONE',  ( 21.05815107556387389, 178.8909823731209485, -125.6365553545643081 ) ) ;
#5600=AXIS2_PLACEMENT_3D ( 'NONE', #2204, #9801, #5211 ) ;
#5601=CARTESIAN_POINT ( 'NONE',  ( 19.90865200055593220, 181.4799304009739558, -122.7714319726113104 ) ) ;
#5606=CARTESIAN_POINT ( 'NONE',  ( -20.00030393798869355, 177.7000510669864184, -124.7934183480526968 ) ) ;
#5632=VERTEX_POINT ( 'NONE', #7522 ) ;
#5636=ORIENTED_EDGE ( 'NONE', *, *, #8356, .F. ) ;
#5647=CARTESIAN_POINT ( 'NONE',  ( 20.00000000000000355, 168.0000000000000000, -124.6807709998038405 ) ) ;
#5651=DIRECTION ( 'NONE',  ( -0.3117078928809505767, -5.319854888938801199E-14, 0.9501779778103246477 ) ) ;
#5664=CARTESIAN_POINT ( 'NONE',  ( 19.97926089986212261, 179.5776042405117323, -126.0284158974866813 ) ) ;
#5665=CIRCLE ( 'NONE', #7244, 11.50000000000003730 ) ;
#5671=TOROIDAL_SURFACE ( 'NONE', #332, 10.00000000000003730, 1.499999999999998002 ) ;
#5672=ORIENTED_EDGE ( 'NONE', *, *, #11302, .T. ) ;
#5676=CARTESIAN_POINT ( 'NONE',  ( -19.91081574664475795, 181.5182364730088125, -122.7941294590836492 ) ) ;
#5677=EDGE_LOOP ( 'NONE', ( #1028, #5535, #9840, #10251, #7438 ) ) ;
#5679=CARTESIAN_POINT ( 'NONE',  ( 28.53314250459842327, 180.2041921146317236, -137.7978499286132319 ) ) ;
#5686=ORIENTED_EDGE ( 'NONE', *, *, #651, .T. ) ;
#5688=EDGE_CURVE ( 'NONE', #7974, #6035, #6954, .T. ) ;
#5691=CARTESIAN_POINT ( 'NONE',  ( 14.74749198504303571, 180.2041921146325762, -184.6327933705058228 ) ) ;
#5693=CARTESIAN_POINT ( 'NONE',  ( 19.94029851291840316, 178.4426130827685029, -123.1320176715209840 ) ) ;
#5697=CARTESIAN_POINT ( 'NONE',  ( -19.99104260667089861, 181.5188412912357308, -125.4148505090950749 ) ) ;
#5701=CARTESIAN_POINT ( 'NONE',  ( 13.32222501832753991, 180.2041921146325762, -184.1652315311844177 ) ) ;
#5745=ORIENTED_EDGE ( 'NONE', *, *, #47, .F. ) ;
#5750=ORIENTED_EDGE ( 'NONE', *, *, #5247, .F. ) ;
#5751=CARTESIAN_POINT ( 'NONE',  ( 19.89219543117309286, 179.2566526312703843, -122.6057988080468277 ) ) ;
#5760=FACE_OUTER_BOUND ( 'NONE', #2705, .T. ) ;
#5763=CIRCLE ( 'NONE', #423, 1.499999999999996447 ) ;
#5771=AXIS2_PLACEMENT_3D ( 'NONE', #4351, #3660, #10090 ) ;
#5779=DIRECTION ( 'NONE',  ( -0.000000000000000000, -1.000000000000000000, -1.757987137413040192E-14 ) ) ;
#5839=ADVANCED_FACE ( 'NONE', ( #6263 ), #2815, .T. ) ;
#5846=EDGE_CURVE ( 'NONE', #9416, #822, #10775, .T. ) ;
#5888=CARTESIAN_POINT ( 'NONE',  ( 20.00183334024216464, 177.6837603104920618, -124.8316880602247068 ) ) ;
#5899=PLANE ( 'NONE',  #2080 ) ;
#5911=CARTESIAN_POINT ( 'NONE',  ( -19.89477560825904234, 178.6155358530109538, -126.7324661926051448 ) ) ;
#5915=EDGE_CURVE ( 'NONE', #9416, #4019, #1627, .T. ) ;
#5926=FACE_OUTER_BOUND ( 'NONE', #4011, .T. ) ;
#5930=SHAPE_REPRESENTATION_RELATIONSHIP ( 'NONE' , 'NONE' ,  #12068, #9120 ) ;
#5946=EDGE_CURVE ( 'NONE', #9851, #20, #5178, .T. ) ;
#5949=ORIENTED_EDGE ( 'NONE', *, *, #9412, .T. ) ;
#5956=CARTESIAN_POINT ( 'NONE',  ( -20.00000000000000000, 182.6968134406616002, -124.6807709998189466 ) ) ;
#5978=AXIS2_PLACEMENT_3D ( 'NONE', #8552, #7806, #7683 ) ;
#5980=CARTESIAN_POINT ( 'NONE',  ( 19.87365484478755917, 180.4904287905548586, -122.4362480607051253 ) ) ;
#5998=CARTESIAN_POINT ( 'NONE',  ( 19.87298152431207399, 180.3898216659918035, -122.4301876295843101 ) ) ;
#6013=CIRCLE ( 'NONE', #11147, 8.500000000000003553 ) ;
#6016=CARTESIAN_POINT ( 'NONE',  ( -19.99999999999999645, 177.7115707886035807, -124.6807709997916334 ) ) ;
#6022=CARTESIAN_POINT ( 'NONE',  ( 7.750278301654327992E-16, 197.0000000000000000, -124.6807709998038405 ) ) ;
#6027=VERTEX_POINT ( 'NONE', #768 ) ;
#6030=CARTESIAN_POINT ( 'NONE',  ( -21.06311735264367613, 179.9260305249855207, -126.4071080971834391 ) ) ;
#6035=VERTEX_POINT ( 'NONE', #12078 ) ;
#6041=DIRECTION ( 'NONE',  ( 1.186840563529527301E-16, -1.000000000000000000, 0.000000000000000000 ) ) ;
#6075=CARTESIAN_POINT ( 'NONE',  ( 19.99507464840871407, 177.7912328150372332, -124.2124546237747609 ) ) ;
#6078=CARTESIAN_POINT ( 'NONE',  ( -19.88197180057522928, 180.9249649884407631, -122.5105553016253737 ) ) ;
#6085=ORIENTED_EDGE ( 'NONE', *, *, #10927, .T. ) ;
#6102=ADVANCED_FACE ( 'NONE', ( #1015 ), #11330, .T. ) ;
#6120=DIRECTION ( 'NONE',  ( -1.000000000000000000, 0.000000000000000000, 0.000000000000000000 ) ) ;
#6126=CARTESIAN_POINT ( 'NONE',  ( -29.03136272649514638, 180.2041921146316668, -134.6807709998038547 ) ) ;
#6130=ORIENTED_EDGE ( 'NONE', *, *, #4346, .T. ) ;
#6133=ORIENTED_EDGE ( 'NONE', *, *, #1036, .F. ) ;
#6134=EDGE_CURVE ( 'NONE', #6278, #4474, #646, .T. ) ;
#6135=CARTESIAN_POINT ( 'NONE',  ( 19.99903954885881063, 178.7487137633693806, -124.2681297334914632 ) ) ;
#6141=ORIENTED_EDGE ( 'NONE', *, *, #1007, .F. ) ;
#6143=CARTESIAN_POINT ( 'NONE',  ( 20.77152989773913916, 180.9696350864299461, -123.5256872951201643 ) ) ;
#6145=ADVANCED_FACE ( 'NONE', ( #248 ), #11310, .F. ) ;
#6157=B_SPLINE_CURVE_WITH_KNOTS ( 'NONE', 3,
 ( #3767, #1739, #6359, #10265, #9273, #8358 ),
 .UNSPECIFIED., .F., .F.,
 ( 4, 2, 4 ),
 ( 9.911001995881279201E-05, 0.0005063982416591003089, 0.0009136864633593878935 ),
 .UNSPECIFIED. ) ;
#6159=CARTESIAN_POINT ( 'NONE',  ( 19.99707640442948886, 182.6412405632554794, -124.2913783979071951 ) ) ;
#6161=CARTESIAN_POINT ( 'NONE',  ( 19.97650381977640066, 180.1919982719466589, -126.1624390054462737 ) ) ;
#6162=AXIS2_PLACEMENT_3D ( 'NONE', #10288, #9367, #4360 ) ;
#6164=TOROIDAL_SURFACE ( 'NONE', #10102, 10.00000000000003730, 1.499999999999998002 ) ;
#6180=DIRECTION ( 'NONE',  ( -0.000000000000000000, -1.000000000000000000, -1.757987137413040192E-14 ) ) ;
#6190=DIRECTION ( 'NONE',  ( -0.05793880415591697725, 0.8576035275428159910, -0.5110374590175372767 ) ) ;
#6198=CARTESIAN_POINT ( 'NONE',  ( -20.77482174596512010, 180.9926187296579201, -123.5402880645762451 ) ) ;
#6217=CARTESIAN_POINT ( 'NONE',  ( 7.750278301654327006E-16, 197.0000000000000000, -124.6807709998038405 ) ) ;
#6218=ORIENTED_EDGE ( 'NONE', *, *, #913, .T. ) ;
#6219=CARTESIAN_POINT ( 'NONE',  ( -20.89767086227280757, 178.8455056537755183, -124.1343435470157743 ) ) ;
#6221=( NAMED_UNIT ( * ) PLANE_ANGLE_UNIT ( ) SI_UNIT ( $, .RADIAN. ) );
#6228=CARTESIAN_POINT ( 'NONE',  ( -21.06614900906485488, 180.8501015263614704, -126.2877667442240153 ) ) ;
#6243=CARTESIAN_POINT ( 'NONE',  ( 20.72176904448479462, 180.0185442467888493, -123.3140496758510949 ) ) ;
#6259=CARTESIAN_POINT ( 'NONE',  ( -19.97808759892263453, 180.7042479906455696, -126.0868659437894053 ) ) ;
#6263=FACE_OUTER_BOUND ( 'NONE', #1898, .T. ) ;
#6273=DIRECTION ( 'NONE',  ( 1.186840563529527301E-16, -1.000000000000000000, 0.000000000000000000 ) ) ;
#6276=CARTESIAN_POINT ( 'NONE',  ( -20.84071877255746230, 179.0301507356313664, -123.8425399495678221 ) ) ;
#6278=VERTEX_POINT ( 'NONE', #2058 ) ;
#6282=CARTESIAN_POINT ( 'NONE',  ( -20.96868743328214890, 181.6918789721509881, -124.6171519127913712 ) ) ;
#6289=CIRCLE ( 'NONE', #156, 19.00000000000000000 ) ;
#6295=CARTESIAN_POINT ( 'NONE',  ( 19.97422267005762109, 181.0592659261928077, -123.4551364493730574 ) ) ;
#6298=EDGE_CURVE ( 'NONE', #6278, #154, #1453, .T. ) ;
#6300=ADVANCED_FACE ( 'NONE', ( #2294 ), #7174, .T. ) ;
#6314=CARTESIAN_POINT ( 'NONE',  ( 20.00000000000000000, 182.6968134406613160, -124.6807709998155076 ) ) ;
#6317=CARTESIAN_POINT ( 'NONE',  ( 20.95930455509759938, 178.7332200987271733, -124.5534165879671207 ) ) ;
#6318=CARTESIAN_POINT ( 'NONE',  ( -19.89655267018000018, 181.8155712312599519, -126.7144533547834016 ) ) ;
#6329=CARTESIAN_POINT ( 'NONE',  ( -19.03136272649511085, 180.2041921146316668, -134.6807709998038547 ) ) ;
#6331=CARTESIAN_POINT ( 'NONE',  ( -20.99127284323103382, 178.6746436565158547, -124.7707208788391284 ) ) ;
#6341=CARTESIAN_POINT ( 'NONE',  ( -19.99337316366387185, 178.8785467397834452, -123.9609963871272100 ) ) ;
#6355=CARTESIAN_POINT ( 'NONE',  ( 19.90865200055529272, 181.4799304009622176, -122.7714319726044607 ) ) ;
#6359=CARTESIAN_POINT ( 'NONE',  ( 21.06505887627893259, 179.6757939811194547, -126.3352607955414442 ) ) ;
#6374=CARTESIAN_POINT ( 'NONE',  ( -20.71964524312745226, 180.3430340654693111, -123.3053720114590703 ) ) ;
#6378=CARTESIAN_POINT ( 'NONE',  ( -21.06252592306710980, 180.0652310508445169, -126.4237660800916245 ) ) ;
#6380=AXIS2_PLACEMENT_3D ( 'NONE', #8336, #7400, #11172 ) ;
#6390=CARTESIAN_POINT ( 'NONE',  ( 19.98008256664037674, 179.4972950632025857, -125.9865773177933477 ) ) ;
#6410=CARTESIAN_POINT ( 'NONE',  ( -19.99589244767088658, 177.7875230617645173, -124.1710050278687447 ) ) ;
#6411=CARTESIAN_POINT ( 'NONE',  ( -20.00000000000000000, 182.6968134406616002, -124.6807709998189466 ) ) ;
#6413=EDGE_LOOP ( 'NONE', ( #7687, #4956, #2925, #7862 ) ) ;
#6423=CARTESIAN_POINT ( 'NONE',  ( 19.98255584530173934, 181.1190424432050179, -125.8592435051848497 ) ) ;
#6444=CARTESIAN_POINT ( 'NONE',  ( -21.06592070232479585, 179.5874863403726636, -126.2949583768656368 ) ) ;
#6454=CARTESIAN_POINT ( 'NONE',  ( 21.06800383392973686, 179.2720088164683432, -126.0983754789175890 ) ) ;
#6457=DIRECTION ( 'NONE',  ( -0.000000000000000000, -1.000000000000000000, -1.757987137413040192E-14 ) ) ;
#6471=CARTESIAN_POINT ( 'NONE',  ( 19.83775307229960916, 179.6904364649550132, -127.2232196724678914 ) ) ;
#6473=CARTESIAN_POINT ( 'NONE',  ( -19.95511007801529857, 178.2536383623800873, -123.3363847648170974 ) ) ;
#6483=CARTESIAN_POINT ( 'NONE',  ( 21.06778670191736325, 181.2627243817148610, -125.9916999785174170 ) ) ;
#6486=CARTESIAN_POINT ( 'NONE',  ( 21.06229719140383594, 181.4525311855803125, -125.7460643626238124 ) ) ;
#6497=LINE ( 'NONE', #750, #2157 ) ;
#6504=CARTESIAN_POINT ( 'NONE',  ( -19.98805534415840057, 182.6507228061688579, -125.3893087125330368 ) ) ;
#6511=DIRECTION ( 'NONE',  ( 1.224646799147353207E-16, 1.453460497224676649E-32, 1.000000000000000000 ) ) ;
#6519=CARTESIAN_POINT ( 'NONE',  ( 19.98895541933857345, 178.9615149398844665, -125.5256490668303400 ) ) ;
#6525=( NAMED_UNIT ( * ) PLANE_ANGLE_UNIT ( ) SI_UNIT ( $, .RADIAN. ) );
#6534=CARTESIAN_POINT ( 'NONE',  ( -20.00030656787924599, 178.6896783452461932, -124.7284307341268459 ) ) ;
#6543=CARTESIAN_POINT ( 'NONE',  ( 19.94162086851303428, 182.2847572333868129, -126.2138291093985742 ) ) ;
#6547=ORIENTED_EDGE ( 'NONE', *, *, #2747, .T. ) ;
#6549=CARTESIAN_POINT ( 'NONE',  ( 4.335549520754014653E-15, 167.0000000000000000, -124.6807709998038405 ) ) ;
#6568=CARTESIAN_POINT ( 'NONE',  ( -19.99960403408873688, 181.6742724572797272, -124.3206507117249799 ) ) ;
#6578=ORIENTED_EDGE ( 'NONE', *, *, #2590, .T. ) ;
#6594=DIRECTION ( 'NONE',  ( 0.000000000000000000, -0.5205506085008965167, -0.8538308169592768726 ) ) ;
#6604=CARTESIAN_POINT ( 'NONE',  ( 19.99606641939810459, 177.7086604316901060, -125.1339395084417276 ) ) ;
#6610=VERTEX_POINT ( 'NONE', #12127 ) ;
#6626=LINE ( 'NONE', #5691, #10996 ) ;
#6654=CARTESIAN_POINT ( 'NONE',  ( 19.97747437608540721, 179.8319032282986143, -126.1164657578071058 ) ) ;
#6674=B_SPLINE_CURVE_WITH_KNOTS ( 'NONE', 3,
 ( #10979, #457, #3364, #4252, #6282, #8022, #11790, #3308, #7086, #10915, #9926, #2445, #6228, #9992, #2507, #5282 ),
 .UNSPECIFIED., .F., .F.,
 ( 4, 2, 2, 2, 2, 2, 2, 4 ),
 ( 0.004753387881373966409, 0.005750299331856708294, 0.006248755057098098753, 0.006747210782339490079, 0.007245666507580881405, 0.007744122232822271863, 0.008242577958063662322, 0.008741033683305053648 ),
 .UNSPECIFIED. ) ;
#6683=CARTESIAN_POINT ( 'NONE',  ( 19.97333794400199025, 179.3704271068745868, -123.4361500813402017 ) ) ;
#6689=DIRECTION ( 'NONE',  ( -0.000000000000000000, -1.000000000000000000, -1.757987137413040192E-14 ) ) ;
#6715=CARTESIAN_POINT ( 'NONE',  ( -19.98540286720293579, 179.1181071172495081, -125.7109378457173676 ) ) ;
#6732=VERTEX_POINT ( 'NONE', #9583 ) ;
#6733=CARTESIAN_POINT ( 'NONE',  ( 20.00000000000011724, 182.6813753181032496, -124.4861612253857004 ) ) ;
#6751=ADVANCED_FACE ( 'NONE', ( #8660 ), #7393, .F. ) ;
#6772=CARTESIAN_POINT ( 'NONE',  ( 19.03136272649511085, 180.2041921146316668, -134.6807709998038547 ) ) ;
#6785=ORIENTED_EDGE ( 'NONE', *, *, #2835, .F. ) ;
#6794=AXIS2_PLACEMENT_3D ( 'NONE', #4388, #10013, #1543 ) ;
#6802=CARTESIAN_POINT ( 'NONE',  ( 19.95730553998325973, 178.2270339500159650, -123.3692462230967521 ) ) ;
#6811=DIRECTION ( 'NONE',  ( 0.000000000000000000, 1.689469820081754479E-14, -1.000000000000000000 ) ) ;
#6818=ORIENTED_EDGE ( 'NONE', *, *, #93, .T. ) ;
#6859=CARTESIAN_POINT ( 'NONE',  ( 20.71964524312746647, 180.2041921146487766, -123.3053720114591414 ) ) ;
#6870=CARTESIAN_POINT ( 'NONE',  ( 19.93152192967729519, 178.5613615780971202, -123.0243173142070816 ) ) ;
#6873=AXIS2_PLACEMENT_3D ( 'NONE', #12062, #6190, #8962 ) ;
#6877=CIRCLE ( 'NONE', #2524, 7.500000000000005329 ) ;
#6882=CARTESIAN_POINT ( 'NONE',  ( -19.97026572922053944, 182.5268623749972505, -125.7890530056691745 ) ) ;
#6897=CARTESIAN_POINT ( 'NONE',  ( -20.00000000000008527, 177.7028087568835417, -124.7912233562835240 ) ) ;
#6899=AXIS2_PLACEMENT_3D ( 'NONE', #6772, #3937, #11479 ) ;
#6904=ORIENTED_EDGE ( 'NONE', *, *, #1187, .F. ) ;
#6908=DIRECTION ( 'NONE',  ( -0.3117078928809505767, -5.319854888938801199E-14, 0.9501779778103246477 ) ) ;
#6910=DIRECTION ( 'NONE',  ( -1.000000000000000000, 0.000000000000000000, 0.000000000000000000 ) ) ;
#6927=CARTESIAN_POINT ( 'NONE',  ( 19.98598762375597460, 179.0443862260074184, -123.7231531907395663 ) ) ;
#6928=EDGE_CURVE ( 'NONE', #3899, #7054, #1397, .T. ) ;
#6929=EDGE_CURVE ( 'NONE', #10270, #2780, #8244, .T. ) ;
#6954=LINE ( 'NONE', #2949, #3202 ) ;
#6974=CARTESIAN_POINT ( 'NONE',  ( 20.89912381907808125, 178.8409046240913085, -124.1420537659444534 ) ) ;
#6996=EDGE_LOOP ( 'NONE', ( #5636, #6218, #1516, #9406 ) ) ;
#6998=CIRCLE ( 'NONE', #1671, 20.00000000000000000 ) ;
#7002=EDGE_CURVE ( 'NONE', #12185, #20, #9953, .T. ) ;
#7004=CARTESIAN_POINT ( 'NONE',  ( 8.937118865183856033E-16, 196.0000000000000000, -124.6807709998038405 ) ) ;
#7010=CARTESIAN_POINT ( 'NONE',  ( 20.00000000000000355, 177.7115707886026144, -124.6807709998038547 ) ) ;
#7018=CYLINDRICAL_SURFACE ( 'NONE', #9552, 7.500000000000005329 ) ;
#7023=CYLINDRICAL_SURFACE ( 'NONE', #1162, 1.500000000000000444 ) ;
#7029=CARTESIAN_POINT ( 'NONE',  ( -19.98684882777175531, 182.5205802027333277, -123.9330515924332161 ) ) ;
#7030=DIRECTION ( 'NONE',  ( -0.9501779778103371932, 0.000000000000000000, 0.3117078928809124960 ) ) ;
#7054=VERTEX_POINT ( 'NONE', #968 ) ;
#7070=AXIS2_PLACEMENT_3D ( 'NONE', #5679, #10316, #1858 ) ;
#7072=CARTESIAN_POINT ( 'NONE',  ( -19.88795444598854445, 178.6948919461029561, -126.7979262391024946 ) ) ;
#7079=CARTESIAN_POINT ( 'NONE',  ( -21.02742354149708603, 178.6868688154197002, -125.1152650341464891 ) ) ;
#7086=CARTESIAN_POINT ( 'NONE',  ( -21.05658410469665043, 181.5474309616008952, -125.5905239331273862 ) ) ;
#7105=ORIENTED_EDGE ( 'NONE', *, *, #651, .F. ) ;
#7122=CARTESIAN_POINT ( 'NONE',  ( -19.91081574664475795, 181.5182364730088125, -122.7941294590836492 ) ) ;
#7170=CARTESIAN_POINT ( 'NONE',  ( 19.88620277217341936, 179.4101426937791075, -122.5498900800241415 ) ) ;
#7171=CARTESIAN_POINT ( 'NONE',  ( -19.92079578072784329, 178.7178626825727576, -122.8973188108788150 ) ) ;
#7174=CYLINDRICAL_SURFACE ( 'NONE', #9155, 20.00000000000000000 ) ;
#7204=CARTESIAN_POINT ( 'NONE',  ( 8.937118865183852088E-16, 196.0000000000000000, -124.6807709998038405 ) ) ;
#7227=CARTESIAN_POINT ( 'NONE',  ( 19.96063188563586266, 182.4486063944580678, -125.9423908938470333 ) ) ;
#7244=AXIS2_PLACEMENT_3D ( 'NONE', #1052, #11362, #11299 ) ;
#7245=CARTESIAN_POINT ( 'NONE',  ( 19.98514591218119563, 182.6308847568197109, -125.4591452170799641 ) ) ;
#7248=DIRECTION ( 'NONE',  ( -1.186840563529527301E-16, 1.000000000000000000, -0.000000000000000000 ) ) ;
#7263=ORIENTED_EDGE ( 'NONE', *, *, #12020, .F. ) ;
#7265=CARTESIAN_POINT ( 'NONE',  ( -21.06224515417718379, 178.9392833470433004, -125.7311303738450050 ) ) ;
#7272=CARTESIAN_POINT ( 'NONE',  ( 20.72444876762976307, 180.4743292376399779, -123.3248083624227291 ) ) ;
#7276=CARTESIAN_POINT ( 'NONE',  ( -19.96345380219486643, 178.1547366163775905, -123.4647820529329323 ) ) ;
#7282=ADVANCED_FACE ( 'NONE', ( #11528 ), #5899, .F. ) ;
#7291=CARTESIAN_POINT ( 'NONE',  ( 19.91016817870376343, 181.9717396535510261, -126.5779665355682084 ) ) ;
#7297=CARTESIAN_POINT ( 'NONE',  ( -19.83159839258490820, 180.4039558769570704, -127.2706957209718581 ) ) ;
#7305=ORIENTED_EDGE ( 'NONE', *, *, #6298, .F. ) ;
#7307=DIRECTION ( 'NONE',  ( -0.05071605604150816737, 0.8431788344085415776, -0.5352357750235388067 ) ) ;
#7315=CARTESIAN_POINT ( 'NONE',  ( -21.06351426534828519, 179.8693486757446465, -126.3917480513811711 ) ) ;
#7322=DIRECTION ( 'NONE',  ( 0.9501779778103313090, 0.000000000000000000, -0.3117078928809301486 ) ) ;
#7325=CARTESIAN_POINT ( 'NONE',  ( 19.98090249381007766, 179.4171559229623654, -125.9448273171951627 ) ) ;
#7332=EDGE_LOOP ( 'NONE', ( #6904, #8815, #6818, #58 ) ) ;
#7337=CARTESIAN_POINT ( 'NONE',  ( -20.80350290787439960, 179.2386340239274887, -123.6703652008354055 ) ) ;
#7351=CARTESIAN_POINT ( 'NONE',  ( 19.99873220238463389, 182.6645275560894106, -124.4081891067125838 ) ) ;
#7354=ORIENTED_EDGE ( 'NONE', *, *, #6298, .T. ) ;
#7368=CARTESIAN_POINT ( 'NONE',  ( -20.77482174596494247, 180.9926187296578348, -123.5402880645763730 ) ) ;
#7372=CARTESIAN_POINT ( 'NONE',  ( -21.06676927307846725, 179.4988070236175588, -126.2505506485803153 ) ) ;
#7381=CARTESIAN_POINT ( 'NONE',  ( 13.32222501832753991, 180.2041921146325762, -184.1652315311844177 ) ) ;
#7393=TOROIDAL_SURFACE ( 'NONE', #2066, 8.500000000000003553, 1.000000000000000000 ) ;
#7400=DIRECTION ( 'NONE',  ( -1.186840563529527301E-16, 1.000000000000000000, 0.000000000000000000 ) ) ;
#7404=CARTESIAN_POINT ( 'NONE',  ( -20.81794809838210369, 179.1660952925545871, -123.7384776798486143 ) ) ;
#7412=CARTESIAN_POINT ( 'NONE',  ( 21.06778026255562253, 181.0036129245391976, -126.2017578805543820 ) ) ;
#7415=CARTESIAN_POINT ( 'NONE',  ( 20.93432090161336490, 181.6310399508034834, -124.3821073715919852 ) ) ;
#7428=CARTESIAN_POINT ( 'NONE',  ( 19.88629874799092789, 181.6918713317650713, -126.8133243770599421 ) ) ;
#7431=ORIENTED_EDGE ( 'NONE', *, *, #1187, .T. ) ;
#7438=ORIENTED_EDGE ( 'NONE', *, *, #3726, .T. ) ;
#7447=ORIENTED_EDGE ( 'NONE', *, *, #5034, .T. ) ;
#7450=FILL_AREA_STYLE_COLOUR ( '', #2880 ) ;
#7465=CARTESIAN_POINT ( 'NONE',  ( -20.94242073755689404, 178.7541906832940128, -124.4271745170988055 ) ) ;
#7474=CIRCLE ( 'NONE', #11810, 1.000000000000000000 ) ;
#7475=CIRCLE ( 'NONE', #8662, 0.9999999999999905631 ) ;
#7476=CARTESIAN_POINT ( 'NONE',  ( 20.82544450079020848, 181.2865457812275736, -123.7704112417842879 ) ) ;
#7479=TOROIDAL_SURFACE ( 'NONE', #9849, 14.02076803445813269, 1.499999999999998002 ) ;
#7488=ORIENTED_EDGE ( 'NONE', *, *, #8441, .F. ) ;
#7491=EDGE_LOOP ( 'NONE', ( #7305, #10789, #12082, #9620 ) ) ;
#7502=B_SPLINE_CURVE_WITH_KNOTS ( 'NONE', 3,
 ( #11738, #3252, #4190, #7029, #11621, #2452, #10919, #5171, #7966, #9812 ),
 .UNSPECIFIED., .F., .F.,
 ( 4, 2, 2, 2, 4 ),
 ( 0.005592014383449837173, 0.006175065507308098722, 0.006758116631166361139, 0.007341167755024623556, 0.007924218878882885106 ),
 .UNSPECIFIED. ) ;
#7516=EDGE_LOOP ( 'NONE', ( #573, #1381, #780, #2100, #765 ) ) ;
#7522=CARTESIAN_POINT ( 'NONE',  ( 19.87268743161337170, 178.9255784920988503, -126.9338343023757290 ) ) ;
#7526=B_SPLINE_CURVE_WITH_KNOTS ( 'NONE', 3,
 ( #4467, #6374, #8311, #12067, #3577, #7368 ),
 .UNSPECIFIED., .F., .F.,
 ( 4, 2, 4 ),
 ( 0.003919203138254567960, 0.004336295509814267618, 0.004753387881373966409 ),
 .UNSPECIFIED. ) ;
#7558=DIRECTION ( 'NONE',  ( 0.3117078928809249860, -1.670400663243698742E-14, 0.9501779778103330854 ) ) ;
#7564=CARTESIAN_POINT ( 'NONE',  ( 21.06598783109611261, 179.0588159534046326, -125.8866071576830734 ) ) ;
#7573=( NAMED_UNIT ( * ) SI_UNIT ( $, .STERADIAN. ) SOLID_ANGLE_UNIT ( ) );
#7582=CARTESIAN_POINT ( 'NONE',  ( -19.94693332216800030, 178.0755435337389656, -126.1424034859261525 ) ) ;
#7617=ORIENTED_EDGE ( 'NONE', *, *, #3448, .F. ) ;
#7618=CARTESIAN_POINT ( 'NONE',  ( -20.98070230502330702, 181.7080454659802342, -124.7060752492303095 ) ) ;
#7633=ORIENTED_EDGE ( 'NONE', *, *, #1258, .T. ) ;
#7639=ORIENTED_EDGE ( 'NONE', *, *, #8739, .F. ) ;
#7646=CARTESIAN_POINT ( 'NONE',  ( -21.01574080354420104, 178.7084824148930693, -125.0322960622685144 ) ) ;
#7665=VERTEX_POINT ( 'NONE', #5523 ) ;
#7668=CARTESIAN_POINT ( 'NONE',  ( 19.94988048130710112, 182.0917278327137865, -123.2593186788816695 ) ) ;
#7674=CIRCLE ( 'NONE', #2350, 1.000000000000000888 ) ;
#7676=CARTESIAN_POINT ( 'NONE',  ( -19.99508847463048156, 181.5683096734331343, -124.0335439678955112 ) ) ;
#7681=ADVANCED_FACE ( 'NONE', ( #11023 ), #1693, .T. ) ;
#7683=DIRECTION ( 'NONE',  ( -1.000000000000000000, -1.186840563529527301E-16, 0.000000000000000000 ) ) ;
#7687=ORIENTED_EDGE ( 'NONE', *, *, #5846, .F. ) ;
#7688=ORIENTED_EDGE ( 'NONE', *, *, #7002, .T. ) ;
#7726=ADVANCED_FACE ( 'NONE', ( #5760 ), #10565, .T. ) ;
#7736=ORIENTED_EDGE ( 'NONE', *, *, #4037, .F. ) ;
#7759=VERTEX_POINT ( 'NONE', #12010 ) ;
#7766=CARTESIAN_POINT ( 'NONE',  ( -19.87519864879852349, 178.8871479037923393, -126.9115732480538838 ) ) ;
#7771=EDGE_LOOP ( 'NONE', ( #10849, #1651, #11405, #4226 ) ) ;
#7798=ADVANCED_FACE ( 'NONE', ( #9971 ), #1745, .T. ) ;
#7806=DIRECTION ( 'NONE',  ( -1.186840563529527301E-16, 1.000000000000000000, -0.000000000000000000 ) ) ;
#7851=CARTESIAN_POINT ( 'NONE',  ( 20.75416591570629876, 179.5558320214803132, -123.4493688440947921 ) ) ;
#7860=ORIENTED_EDGE ( 'NONE', *, *, #1645, .F. ) ;
#7862=ORIENTED_EDGE ( 'NONE', *, *, #4202, .T. ) ;
#7863=CARTESIAN_POINT ( 'NONE',  ( 19.99397847396136996, 178.8651426120512724, -123.9853605248128474 ) ) ;
#7878=CARTESIAN_POINT ( 'NONE',  ( -19.98117600975061592, 182.6057245623286462, -125.5759384559340077 ) ) ;
#7886=( BOUNDED_SURFACE ( )  B_SPLINE_SURFACE ( 3, 2, ( 
 ( #6355, #6295, #8155 ),
 ( #4383, #1854, #3698 ),
 ( #10065, #1596, #7476 ),
 ( #8353, #1661, #9073 ),
 ( #5358, #4644, #10193 ),
 ( #11254, #3560, #3630 ),
 ( #870, #1733, #7415 ),
 ( #7351, #9134, #11056 ),
 ( #5421, #608, #11923 ),
 ( #11191, #4513, #2582 ),
 ( #3444, #674, #4449 ),
 ( #11122, #8421, #12183 ),
 ( #10994, #11985, #2713 ),
 ( #1791, #8225, #5493 ),
 ( #7227, #2779, #10258 ),
 ( #6543, #10126, #6486 ),
 ( #8292, #2521, #3502 ),
 ( #7291, #9200, #12048 ),
 ( #2647, #6423, #9266 ),
 ( #808, #4580, #12117 ),
 ( #5556, #10313, #9330 ),
 ( #10797, #2334, #5222 ),
 ( #459, #4254, #8023 ),
 ( #527, #6161, #9927 ),
 ( #10360, #3544, #11173 ),
 ( #6471, #30, #11105 ),
 ( #9498, #6654, #1040 ),
 ( #8466, #9379, #9314 ),
 ( #1714, #5664, #10243 ),
 ( #5541, #11350, #5473 ) ),
 .UNSPECIFIED., .F., .F., .F. ) 
 B_SPLINE_SURFACE_WITH_KNOTS ( ( 4, 2, 2, 2, 2, 2, 2, 2, 2, 2, 2, 2, 2, 2, 4 ),
 ( 3, 3 ),
 ( 0.007889744914357701283, 0.008875963028655821374, 0.009369072085804883154, 0.009862181142953943200, 0.01035529020010300325, 0.01084839925725206503, 0.01134150831440112507, 0.01183461737155018512, 0.01232772642869924516, 0.01282083548584830521, 0.01380705360014642703, 0.01430016265729548708, 0.01479327171444454886, 0.01528638077159360890, 0.01577948982874266895 ),
 ( 0.000000000000000000, 1.000000000000000000 ),
 .UNSPECIFIED. ) 
 GEOMETRIC_REPRESENTATION_ITEM ( )  RATIONAL_B_SPLINE_SURFACE ( (
 ( 1.000000000000000000, 0.7788034628477763510, 1.000000000000000000),
 ( 1.000000000000000000, 0.7721230128607156074, 1.000000000000000000),
 ( 1.000000000000000000, 0.7637060791568476281, 1.000000000000000000),
 ( 1.000000000000000000, 0.7496516620472627457, 1.000000000000000000),
 ( 1.000000000000000000, 0.7447560477940591284, 1.000000000000000000),
 ( 1.000000000000000000, 0.7349957282090778810, 1.000000000000000000),
 ( 1.000000000000000000, 0.7300720695073790178, 1.000000000000000000),
 ( 1.000000000000000000, 0.7203457075533885590, 1.000000000000000000),
 ( 1.000000000000000000, 0.7156722358407558993, 1.000000000000000000),
 ( 1.000000000000000000, 0.7067788860353876323, 1.000000000000000000),
 ( 1.000000000000000000, 0.7025175898284636844, 1.000000000000000000),
 ( 1.000000000000000000, 0.6947521172562991509, 1.000000000000000000),
 ( 1.000000000000000000, 0.6912534286752571866, 1.000000000000000000),
 ( 1.000000000000000000, 0.6849888440347751128, 1.000000000000000000),
 ( 1.000000000000000000, 0.6822120470311171525, 1.000000000000000000),
 ( 1.000000000000000000, 0.6775429675546015273, 1.000000000000000000),
 ( 1.000000000000000000, 0.6756152869907889880, 1.000000000000000000),
 ( 1.000000000000000000, 0.6724212228960821935, 1.000000000000000000),
 ( 1.000000000000000000, 0.6711767660106030542, 1.000000000000000000),
 ( 1.000000000000000000, 0.6682954301978540901, 1.000000000000000000),
 ( 1.000000000000000000, 0.6674300803999402287, 1.000000000000000000),
 ( 1.000000000000000000, 0.6667725974591163229, 1.000000000000000000),
 ( 1.000000000000000000, 0.6666584258004638608, 1.000000000000000000),
 ( 1.000000000000000000, 0.6665746734483880553, 1.000000000000000000),
 ( 1.000000000000000000, 0.6666022109305942411, 1.000000000000000000),
 ( 1.000000000000000000, 0.6668181847376934979, 1.000000000000000000),
 ( 1.000000000000000000, 0.6670097042269241827, 1.000000000000000000),
 ( 1.000000000000000000, 0.6676556552395226385, 1.000000000000000000),
 ( 1.000000000000000000, 0.6681120711471668638, 1.000000000000000000),
 ( 1.000000000000000000, 0.6687969305523246977, 1.000000000000000000) ) ) 
 REPRESENTATION_ITEM ( '' )  SURFACE ( )  );
#7900=EDGE_LOOP ( 'NONE', ( #927, #11497, #3578, #2584 ) ) ;
#7905=CARTESIAN_POINT ( 'NONE',  ( 19.89852930574608791, 181.2981474642644741, -122.6658827718632949 ) ) ;
#7927=DIRECTION ( 'NONE',  ( 0.000000000000000000, -1.000000000000000000, -1.850371707708592551E-14 ) ) ;
#7955=DIRECTION ( 'NONE',  ( 1.000000000000000000, 0.000000000000000000, 0.000000000000000000 ) ) ;
#7966=CARTESIAN_POINT ( 'NONE',  ( -19.92026566182175884, 181.6832013291224541, -122.8938598614162174 ) ) ;
#7974=VERTEX_POINT ( 'NONE', #5647 ) ;
#7981=CARTESIAN_POINT ( 'NONE',  ( 20.71882545568003664, 180.2153781204678182, -123.3020207091857401 ) ) ;
#7984=VECTOR ( 'NONE', #1815, 1000.000000000000000 ) ;
#8004=AXIS2_PLACEMENT_3D ( 'NONE', #7381, #3530, #7322 ) ;
#8007=CARTESIAN_POINT ( 'NONE',  ( 4.216865464401061553E-15, 168.0000000000000000, -124.6807709998038405 ) ) ;
#8011=CARTESIAN_POINT ( 'NONE',  ( -19.98192996636583274, 177.7975057939641772, -125.5577353981673099 ) ) ;
#8013=B_SPLINE_CURVE_WITH_KNOTS ( 'NONE', 3,
 ( #4690, #8465, #5404, #7272, #8274, #3683 ),
 .UNSPECIFIED., .F., .F.,
 ( 4, 2, 4 ),
 ( 0.004972348860735044569, 0.005379997031218691772, 0.005787645201702338975 ),
 .UNSPECIFIED. ) ;
#8016=CARTESIAN_POINT ( 'NONE',  ( -21.06809339192879449, 179.1479816184320271, -125.9940397287191161 ) ) ;
#8022=CARTESIAN_POINT ( 'NONE',  ( -21.00772343926389141, 181.7109892249738436, -124.9456595701584831 ) ) ;
#8023=CARTESIAN_POINT ( 'NONE',  ( 21.06267721941133786, 180.3886733041073001, -126.4187213689463505 ) ) ;
#8024=CARTESIAN_POINT ( 'NONE',  ( 19.87738559348426648, 180.7004044570965675, -122.4687948322674345 ) ) ;
#8026=CARTESIAN_POINT ( 'NONE',  ( -20.00000000000000000, 196.0000000000000000, -124.6807709998038405 ) ) ;
#8051=DIRECTION ( 'NONE',  ( 0.000000000000000000, 0.5359254506312245425, 0.8442653086356912695 ) ) ;
#8060=DIRECTION ( 'NONE',  ( -1.186840563529527301E-16, 1.000000000000000000, -0.000000000000000000 ) ) ;
#8067=AXIS2_PLACEMENT_3D ( 'NONE', #6126, #9893, #372 ) ;
#8078=ORIENTED_EDGE ( 'NONE', *, *, #4663, .F. ) ;
#8087=DIRECTION ( 'NONE',  ( -0.3117078928809153826, -1.979053562451413181E-14, -0.9501779778103363050 ) ) ;
#8100=CARTESIAN_POINT ( 'NONE',  ( -19.99524239788497226, 182.6919990222411343, -125.1313804517642581 ) ) ;
#8115=CARTESIAN_POINT ( 'NONE',  ( -19.97651234637680417, 180.1670482320588178, -126.1620355637344346 ) ) ;
#8121=AXIS2_PLACEMENT_3D ( 'NONE', #6329, #9301, #10967 ) ;
#8122=DIRECTION ( 'NONE',  ( -1.000000000000000000, -1.186840563529527301E-16, 0.000000000000000000 ) ) ;
#8133=DIRECTION ( 'NONE',  ( 1.000000000000000000, 0.000000000000000000, 0.000000000000000000 ) ) ;
#8138=DIRECTION ( 'NONE',  ( 0.000000000000000000, -0.5273567215051647716, -0.8496439773713011512 ) ) ;
#8155=CARTESIAN_POINT ( 'NONE',  ( 20.77152989773915692, 180.9696350864299461, -123.5256872951201217 ) ) ;
#8159=CARTESIAN_POINT ( 'NONE',  ( 20.77152989774015168, 180.9696350864370231, -123.5256872951244986 ) ) ;
#8177=ORIENTED_EDGE ( 'NONE', *, *, #2368, .F. ) ;
#8188=CARTESIAN_POINT ( 'NONE',  ( -21.06240745282759974, 180.0655816779955956, -126.4269926335278882 ) ) ;
#8189=CARTESIAN_POINT ( 'NONE',  ( 20.86817559351791473, 181.4710734879092797, -123.9731132673169185 ) ) ;
#8190=EDGE_CURVE ( 'NONE', #5632, #505, #552, .T. ) ;
#8193=EDGE_CURVE ( 'NONE', #7665, #8550, #7475, .T. ) ;
#8207=DIRECTION ( 'NONE',  ( 0.000000000000000000, -0.000000000000000000, -1.000000000000000000 ) ) ;
#8211=CARTESIAN_POINT ( 'NONE',  ( -19.89048104400029260, 179.2983987876859544, -122.5895104425266879 ) ) ;
#8225=CARTESIAN_POINT ( 'NONE',  ( 19.99143708932781749, 181.5311400647427149, -125.3935307427316701 ) ) ;
#8230=CARTESIAN_POINT ( 'NONE',  ( -19.87204390493025130, 180.1031888591127768, -122.4220199087763064 ) ) ;
#8244=B_SPLINE_CURVE_WITH_KNOTS ( 'NONE', 3,
 ( #713, #11845, #8016, #7265, #587, #7079, #6331, #6219, #6276, #11032, #3478, #4364, #3357, #3089 ),
 .UNSPECIFIED., .F., .F.,
 ( 4, 2, 2, 2, 2, 2, 4 ),
 ( 0.009574516480326976040, 0.01007331370637661733, 0.01057211093242625688, 0.01156970538452561578, 0.01256729983662497468, 0.01306609706267465414, 0.01356489428872433359 ),
 .UNSPECIFIED. ) ;
#8259=DIRECTION ( 'NONE',  ( -1.000000000000000000, 0.000000000000000000, 0.000000000000000000 ) ) ;
#8274=CARTESIAN_POINT ( 'NONE',  ( 20.71964524312787148, 180.3384025927469736, -123.3053720114607614 ) ) ;
#8292=CARTESIAN_POINT ( 'NONE',  ( 19.93132511079140556, 182.1895273313274117, -126.3410201175955478 ) ) ;
#8311=CARTESIAN_POINT ( 'NONE',  ( -20.72478464386518482, 180.4834696826887921, -123.3261552949825131 ) ) ;
#8314=CARTESIAN_POINT ( 'NONE',  ( -19.90725264551396378, 181.9394096378942720, -126.6082001725200570 ) ) ;
#8319=CARTESIAN_POINT ( 'NONE',  ( -19.00000000000000000, 196.0000000000000000, -124.6807709998038405 ) ) ;
#8325=DIRECTION ( 'NONE',  ( -0.000000000000000000, -1.000000000000000000, -1.757987137413040192E-14 ) ) ;
#8332=( LENGTH_UNIT ( ) NAMED_UNIT ( * ) SI_UNIT ( .MILLI., .METRE. ) );
#8336=CARTESIAN_POINT ( 'NONE',  ( 2.510525938252073693E-14, -7.999999999999979572, -124.6807709998038405 ) ) ;
#8340=CARTESIAN_POINT ( 'NONE',  ( -19.87629508054677174, 179.7764057819409516, -122.4594234116466538 ) ) ;
#8349=DIRECTION ( 'NONE',  ( -1.000000000000000000, 0.000000000000000000, 0.000000000000000000 ) ) ;
#8350=CARTESIAN_POINT ( 'NONE',  ( 20.00000000000000355, 177.7115707886026144, -124.6807709998038547 ) ) ;
#8353=CARTESIAN_POINT ( 'NONE',  ( 19.96746008154850927, 182.3013212999341590, -123.5332635133612200 ) ) ;
#8356=EDGE_CURVE ( 'NONE', #9220, #2139, #9036, .T. ) ;
#8358=CARTESIAN_POINT ( 'NONE',  ( 21.06240745282767435, 180.2041921146315246, -126.4269926335259413 ) ) ;
#8362=( BOUNDED_SURFACE ( )  B_SPLINE_SURFACE ( 3, 2, ( 
 ( #773, #6390, #3791 ),
 ( #3532, #7325, #2809 ),
 ( #11156, #11090, #6454 ),
 ( #12154, #10162, #1695 ),
 ( #2682, #10227, #7564 ),
 ( #9233, #3669, #4547 ),
 ( #2749, #6519, #5587 ),
 ( #10286, #1826, #909 ),
 ( #4841, #3856, #8685 ),
 ( #3050, #78, #2129 ),
 ( #5888, #8738, #255 ),
 ( #4046, #10829, #6317 ),
 ( #6075, #9842, #2367 ),
 ( #10884, #6135, #1378 ),
 ( #5141, #2482, #11142 ),
 ( #3901, #7863, #1006 ),
 ( #6802, #9650, #2049 ),
 ( #5693, #6927, #4775 ),
 ( #6870, #11445, #3841 ),
 ( #10638, #126, #9711 ),
 ( #11383, #6683, #1993 ),
 ( #5751, #1071, #8951 ),
 ( #7170, #416, #11809 ),
 ( #10011, #3326, #10936 ),
 ( #10868, #2467, #6243 ),
 ( #4205, #5240, #7981 ),
 ( #5998, #11752, #2404 ),
 ( #9075, #9012, #9766 ),
 ( #610, #547, #3447 ),
 ( #4386, #1310, #8159 ) ),
 .UNSPECIFIED., .F., .F., .F. ) 
 B_SPLINE_SURFACE_WITH_KNOTS ( ( 4, 2, 2, 2, 2, 2, 2, 2, 2, 2, 2, 2, 2, 2, 4 ),
 ( 3, 3 ),
 ( 0.000000000000000000, 0.0004931090571482092720, 0.0009862181142964185441, 0.001479327171444627925, 0.001972436228592837088, 0.002958654342889255849, 0.003451763400037465013, 0.003944872457185674176, 0.004437981514333883340, 0.004931090571482093371, 0.005424199628630302535, 0.005917308685778511698, 0.006410417742926720862, 0.006903526800074930025, 0.007889744914371348353 ),
 ( 0.000000000000000000, 1.000000000000000000 ),
 .UNSPECIFIED. ) 
 GEOMETRIC_REPRESENTATION_ITEM ( )  RATIONAL_B_SPLINE_SURFACE ( (
 ( 1.000000000000000000, 0.6687969305523246977, 1.000000000000000000),
 ( 1.000000000000000000, 0.6694841494169265772, 1.000000000000000000),
 ( 1.000000000000000000, 0.6703808696174045068, 1.000000000000000000),
 ( 1.000000000000000000, 0.6727883736869240128, 1.000000000000000000),
 ( 1.000000000000000000, 0.6743212217357245075, 1.000000000000000000),
 ( 1.000000000000000000, 0.6781193367449044329, 1.000000000000000000),
 ( 1.000000000000000000, 0.6803721377959787153, 1.000000000000000000),
 ( 1.000000000000000000, 0.6857220711556456516, 1.000000000000000000),
 ( 1.000000000000000000, 0.6888414615222259174, 1.000000000000000000),
 ( 1.000000000000000000, 0.6991960670388784882, 1.000000000000000000),
 ( 1.000000000000000000, 0.7077353972677926652, 1.000000000000000000),
 ( 1.000000000000000000, 0.7216195274859381614, 1.000000000000000000),
 ( 1.000000000000000000, 0.7264787526967504405, 1.000000000000000000),
 ( 1.000000000000000000, 0.7363107972878868424, 1.000000000000000000),
 ( 1.000000000000000000, 0.7412133880338421799, 1.000000000000000000),
 ( 1.000000000000000000, 0.7508641489171165029, 1.000000000000000000),
 ( 1.000000000000000000, 0.7556596050786191787, 1.000000000000000000),
 ( 1.000000000000000000, 0.7646032520811554267, 1.000000000000000000),
 ( 1.000000000000000000, 0.7687769290552097790, 1.000000000000000000),
 ( 1.000000000000000000, 0.7763903678017805010, 1.000000000000000000),
 ( 1.000000000000000000, 0.7798239438996181772, 1.000000000000000000),
 ( 1.000000000000000000, 0.7855160016894544572, 1.000000000000000000),
 ( 1.000000000000000000, 0.7878236855009348449, 1.000000000000000000),
 ( 1.000000000000000000, 0.7912368103514670903, 1.000000000000000000),
 ( 1.000000000000000000, 0.7922947285227288639, 1.000000000000000000),
 ( 1.000000000000000000, 0.7930773382062819010, 1.000000000000000000),
 ( 1.000000000000000000, 0.7928003068872482295, 1.000000000000000000),
 ( 1.000000000000000000, 0.7899630766598022547, 1.000000000000000000),
 ( 1.000000000000000000, 0.7854601384747740278, 1.000000000000000000),
 ( 1.000000000000000000, 0.7788034628475056786, 1.000000000000000000) ) ) 
 REPRESENTATION_ITEM ( '' )  SURFACE ( )  );
#8371=CARTESIAN_POINT ( 'NONE',  ( 19.86104407927658144, 181.3041390551380800, -127.0369522072293194 ) ) ;
#8373=VERTEX_POINT ( 'NONE', #2399 ) ;
#8374=CARTESIAN_POINT ( 'NONE',  ( -19.98868386570119782, 182.5424741720831889, -123.9930727067244902 ) ) ;
#8388=CIRCLE ( 'NONE', #2446, 7.500000000000005329 ) ;
#8410=CARTESIAN_POINT ( 'NONE',  ( -20.72447511889459904, 179.9475203146823787, -123.3250521315598718 ) ) ;
#8421=CARTESIAN_POINT ( 'NONE',  ( 19.99569434005708857, 181.6422274730699371, -125.1461840823352816 ) ) ;
#8437=CARTESIAN_POINT ( 'NONE',  ( 19.94501782540249124, 182.3171294987543263, -126.1758857494099146 ) ) ;
#8441=EDGE_CURVE ( 'NONE', #5632, #6035, #4250, .T. ) ;
#8443=CARTESIAN_POINT ( 'NONE',  ( -21.03188327321321083, 181.6721105287138300, -125.2135271367785236 ) ) ;
#8465=CARTESIAN_POINT ( 'NONE',  ( 20.75549287943134402, 180.8556829965724546, -123.4547523536870557 ) ) ;
#8466=CARTESIAN_POINT ( 'NONE',  ( 19.85548708303895893, 179.2177006722742192, -127.0812667107773564 ) ) ;
#8480=ORIENTED_EDGE ( 'NONE', *, *, #11375, .T. ) ;
#8497=CARTESIAN_POINT ( 'NONE',  ( -19.94556339419311186, 182.0394078756253293, -123.1838850670707188 ) ) ;
#8534=DIRECTION ( 'NONE',  ( -0.000000000000000000, -1.000000000000000000, -1.757987137413040192E-14 ) ) ;
#8544=ORIENTED_EDGE ( 'NONE', *, *, #740, .T. ) ;
#8550=VERTEX_POINT ( 'NONE', #10257 ) ;
#8552=CARTESIAN_POINT ( 'NONE',  ( 4.454233577106967753E-15, 166.0000000000000000, -124.6807709998038405 ) ) ;
#8567=ORIENTED_EDGE ( 'NONE', *, *, #8739, .T. ) ;
#8576=CARTESIAN_POINT ( 'NONE',  ( -21.02500011264404023, 178.7212721744384396, -125.1324667871970036 ) ) ;
#8584=CARTESIAN_POINT ( 'NONE',  ( 19.87268743161337170, 178.9255784920988503, -126.9338343023757290 ) ) ;
#8586=EDGE_CURVE ( 'NONE', #10417, #7974, #10427, .T. ) ;
#8612=CARTESIAN_POINT ( 'NONE',  ( -19.03136272649511085, 180.2041921146316668, -134.6807709998038547 ) ) ;
#8636=PRODUCT_DEFINITION_CONTEXT ( 'detailed design', #4235, 'design' ) ;
#8639=CARTESIAN_POINT ( 'NONE',  ( -21.06687908627628403, 179.1075766945866121, -125.9428570876586804 ) ) ;
#8640=EDGE_CURVE ( 'NONE', #11203, #10417, #2529, .T. ) ;
#8660=FACE_OUTER_BOUND ( 'NONE', #1085, .T. ) ;
#8662=AXIS2_PLACEMENT_3D ( 'NONE', #491, #7307, #8051 ) ;
#8685=CARTESIAN_POINT ( 'NONE',  ( 21.04250863801212290, 178.7733595539146734, -125.3557961042217386 ) ) ;
#8690=ORIENTED_EDGE ( 'NONE', *, *, #11312, .F. ) ;
#8698=CARTESIAN_POINT ( 'NONE',  ( 4.335549520754014653E-15, 167.0000000000000000, -124.6807709998038405 ) ) ;
#8700=CARTESIAN_POINT ( 'NONE',  ( -19.97345815004482716, 177.8596483071499108, -125.7207219634393311 ) ) ;
#8706=DIRECTION ( 'NONE',  ( -1.224646799147353207E-16, -1.453460497224676649E-32, 1.000000000000000000 ) ) ;
#8738=CARTESIAN_POINT ( 'NONE',  ( 19.99986396686996670, 178.6891417861111790, -124.8519595561770359 ) ) ;
#8739=EDGE_CURVE ( 'NONE', #569, #8373, #3509, .T. ) ;
#8741=CARTESIAN_POINT ( 'NONE',  ( -19.99905741042869423, 182.7066083885001149, -124.9054265645020365 ) ) ;
#8742=CARTESIAN_POINT ( 'NONE',  ( -19.96332333990081764, 180.6948238841417265, -123.2561630805032848 ) ) ;
#8750=PRODUCT_CONTEXT ( 'NONE', #10713, 'mechanical' ) ;
#8758=CARTESIAN_POINT ( 'NONE',  ( -19.88457985033570097, 178.7457540148283499, -126.8279919963933509 ) ) ;
#8762=ORIENTED_EDGE ( 'NONE', *, *, #8441, .T. ) ;
#8773=DIRECTION ( 'NONE',  ( -1.186840563529527301E-16, 1.000000000000000000, -0.000000000000000000 ) ) ;
#8775=CARTESIAN_POINT ( 'NONE',  ( 6.500000000000030198, -7.999999999999979572, -124.6807709998038405 ) ) ;
#8779=CARTESIAN_POINT ( 'NONE',  ( 19.03136272649511085, 180.2041921146316668, -134.6807709998038547 ) ) ;
#8806=DIRECTION ( 'NONE',  ( 0.9501779778103254248, 0.000000000000000000, 0.3117078928809486338 ) ) ;
#8815=ORIENTED_EDGE ( 'NONE', *, *, #6928, .T. ) ;
#8816=DIRECTION ( 'NONE',  ( -1.000000000000000000, 0.000000000000000000, 0.000000000000000000 ) ) ;
#8824=DIRECTION ( 'NONE',  ( 1.000000000000000000, 0.000000000000000000, 0.000000000000000000 ) ) ;
#8840=EDGE_LOOP ( 'NONE', ( #9331, #8567 ) ) ;
#8850=CIRCLE ( 'NONE', #3122, 1.000000000000005773 ) ;
#8865=DIRECTION ( 'NONE',  ( -1.000000000000000000, 0.000000000000000000, 0.000000000000000000 ) ) ;
#8904=DIRECTION ( 'NONE',  ( 1.000000000000000000, 0.000000000000000000, 0.000000000000000000 ) ) ;
#8913=CARTESIAN_POINT ( 'NONE',  ( 20.81144718909768798, 181.2532700293135974, -123.7022494633698102 ) ) ;
#8929=CARTESIAN_POINT ( 'NONE',  ( 19.97592758413811254, 178.0092090781685670, -123.6846453938936747 ) ) ;
#8936=CARTESIAN_POINT ( 'NONE',  ( 21.05748054007814218, 178.8679675183088875, -125.6049322330816409 ) ) ;
#8941=DIRECTION ( 'NONE',  ( -0.000000000000000000, -1.000000000000000000, -1.757987137413040192E-14 ) ) ;
#8951=CARTESIAN_POINT ( 'NONE',  ( 20.74704732419727193, 179.6356684247163571, -123.4191576945881224 ) ) ;
#8962=DIRECTION ( 'NONE',  ( 0.000000000000000000, 0.5118973767283547804, 0.8590466085717518574 ) ) ;
#8968=CIRCLE ( 'NONE', #4055, 8.500000000000035527 ) ;
#8969=CARTESIAN_POINT ( 'NONE',  ( -19.98030737385957423, 179.4757119253121402, -125.9751133749524712 ) ) ;
#8970=DIRECTION ( 'NONE',  ( -1.186840563529527301E-16, 1.000000000000000000, -0.000000000000000000 ) ) ;
#8994=CARTESIAN_POINT ( 'NONE',  ( -21.06729583384051097, 179.4139655881280078, -126.1965993184190040 ) ) ;
#8998=EDGE_CURVE ( 'NONE', #2717, #20, #6497, .T. ) ;
#9012=CARTESIAN_POINT ( 'NONE',  ( 19.96273514930160431, 180.6655135177861382, -123.2465523723562910 ) ) ;
#9018=DIRECTION ( 'NONE',  ( 0.000000000000000000, -1.757987137413040192E-14, 1.000000000000000000 ) ) ;
#9027=CARTESIAN_POINT ( 'NONE',  ( -19.97946372138042648, 179.5552863838666156, -126.0181968814597582 ) ) ;
#9028=VERTEX_POINT ( 'NONE', #9342 ) ;
#9036=CIRCLE ( 'NONE', #5275, 6.500000000000005329 ) ;
#9037=DIRECTION ( 'NONE',  ( -1.000000000000000000, 0.000000000000000000, 0.000000000000000000 ) ) ;
#9048=CARTESIAN_POINT ( 'NONE',  ( 0.000000000000000000, 0.000000000000000000, 0.000000000000000000 ) ) ;
#9065=CIRCLE ( 'NONE', #11839, 8.500000000000035527 ) ;
#9073=CARTESIAN_POINT ( 'NONE',  ( 20.87244046619806070, 181.4624696265101704, -124.0161187626494126 ) ) ;
#9075=CARTESIAN_POINT ( 'NONE',  ( 19.88060343642096583, 180.8815710988893954, -122.4981836151635264 ) ) ;
#9087=EDGE_CURVE ( 'NONE', #559, #12185, #7674, .T. ) ;
#9090=CARTESIAN_POINT ( 'NONE',  ( -19.83289927702564626, 180.4664674243214506, -127.2607214279775008 ) ) ;
#9111=DIRECTION ( 'NONE',  ( 1.186840563529527301E-16, -1.000000000000000000, 0.000000000000000000 ) ) ;
#9118=FACE_OUTER_BOUND ( 'NONE', #1202, .T. ) ;
#9120=ADVANCED_BREP_SHAPE_REPRESENTATION ( '', ( #12079, #11957 ), #3662 ) ;
#9122=CARTESIAN_POINT ( 'NONE',  ( -19.96691528312132036, 179.5908022299374522, -123.3171134976379761 ) ) ;
#9134=CARTESIAN_POINT ( 'NONE',  ( 20.00075211776240991, 181.7166608263125056, -124.5881005502433823 ) ) ;
#9138=CARTESIAN_POINT ( 'NONE',  ( -19.87400029745858987, 179.8933018207857515, -122.4388957686745272 ) ) ;
#9151=CARTESIAN_POINT ( 'NONE',  ( 19.84972815362622001, 179.3291729170307462, -127.1285282547103890 ) ) ;
#9153=AXIS2_PLACEMENT_3D ( 'NONE', #12173, #2771, #4564 ) ;
#9155=AXIS2_PLACEMENT_3D ( 'NONE', #3211, #3332, #1430 ) ;
#9156=CARTESIAN_POINT ( 'NONE',  ( -19.98332493385930420, 181.1706761403379744, -125.8191529278201131 ) ) ;
#9183=DIRECTION ( 'NONE',  ( -0.05908736525064870598, -0.8481594924192722429, 0.5264353319134452702 ) ) ;
#9195=DIRECTION ( 'NONE',  ( -1.000000000000000000, -1.186840563529527301E-16, 0.000000000000000000 ) ) ;
#9200=CARTESIAN_POINT ( 'NONE',  ( 19.98362395802042712, 181.1895308572829890, -125.8035797126588733 ) ) ;
#9204=AXIS2_PLACEMENT_3D ( 'NONE', #4225, #3399, #10035 ) ;
#9206=DIRECTION ( 'NONE',  ( 1.186840563529527301E-16, -1.000000000000000000, 0.000000000000000000 ) ) ;
#9220=VERTEX_POINT ( 'NONE', #8775 ) ;
#9221=CARTESIAN_POINT ( 'NONE',  ( -21.06792119228306603, 181.1710195846050340, -126.0693529377697786 ) ) ;
#9233=CARTESIAN_POINT ( 'NONE',  ( 19.94423941549897705, 178.0993878143254676, -126.1785714357287702 ) ) ;
#9235=FACE_OUTER_BOUND ( 'NONE', #942, .T. ) ;
#9247=CARTESIAN_POINT ( 'NONE',  ( -20.86895858123844860, 178.8871479037923393, -127.0231133604663682 ) ) ;
#9252=CARTESIAN_POINT ( 'NONE',  ( -19.95962463553759392, 180.3623627298850067, -123.1966106898677964 ) ) ;
#9260=CARTESIAN_POINT ( 'NONE',  ( 20.00000000000000355, 167.0000000000000000, -124.6807709998038405 ) ) ;
#9262=CARTESIAN_POINT ( 'NONE',  ( 21.06240745282767435, 180.3710338094945200, -126.4269926335259129 ) ) ;
#9266=CARTESIAN_POINT ( 'NONE',  ( 21.06786593334110336, 181.1916812352232853, -126.0511736859032936 ) ) ;
#9271=CIRCLE ( 'NONE', #176, 1.499999999999996447 ) ;
#9273=CARTESIAN_POINT ( 'NONE',  ( 21.06240745282767435, 180.0702511251071485, -126.4269926335259413 ) ) ;
#9280=ORIENTED_EDGE ( 'NONE', *, *, #1036, .T. ) ;
#9286=CARTESIAN_POINT ( 'NONE',  ( 19.99610756949845225, 182.6998913380727743, -125.1317435956655117 ) ) ;
#9290=CARTESIAN_POINT ( 'NONE',  ( -19.98563867331158406, 181.3023397240705776, -125.6985981901809453 ) ) ;
#9292=ORIENTED_EDGE ( 'NONE', *, *, #5688, .T. ) ;
#9301=DIRECTION ( 'NONE',  ( -0.000000000000000000, -1.000000000000000000, -1.757987137413040192E-14 ) ) ;
#9314=CARTESIAN_POINT ( 'NONE',  ( 21.06569119078285013, 179.6122972493173222, -126.3061156060180963 ) ) ;
#9316=CARTESIAN_POINT ( 'NONE',  ( -19.03136272649511085, 180.2041921146316668, -134.6807709998038547 ) ) ;
#9317=CARTESIAN_POINT ( 'NONE',  ( -19.98204207764186791, 179.1370916267982523, -123.6234561704243475 ) ) ;
#9327=CARTESIAN_POINT ( 'NONE',  ( 19.88538568419372154, 178.7282225113628726, -126.8218319435565604 ) ) ;
#9330=CARTESIAN_POINT ( 'NONE',  ( 21.06533532366276162, 180.7746266989912272, -126.3260595342268715 ) ) ;
#9331=ORIENTED_EDGE ( 'NONE', *, *, #11060, .T. ) ;
#9335=DIRECTION ( 'NONE',  ( -1.000000000000000000, 0.000000000000000000, 0.000000000000000000 ) ) ;
#9342=CARTESIAN_POINT ( 'NONE',  ( 29.95840947131252108, 180.2041921146317520, -138.2654117679341539 ) ) ;
#9343=ADVANCED_FACE ( 'NONE', ( #1728, #2576 ), #5486, .F. ) ;
#9351=CARTESIAN_POINT ( 'NONE',  ( -19.99699311396506118, 181.6109172643918157, -124.1290590095319430 ) ) ;
#9367=DIRECTION ( 'NONE',  ( -1.224646799147353207E-16, -1.453460497224676649E-32, 1.000000000000000000 ) ) ;
#9379=CARTESIAN_POINT ( 'NONE',  ( 19.97857452415077972, 179.6604161890264493, -126.0626113202902587 ) ) ;
#9383=CARTESIAN_POINT ( 'NONE',  ( -19.99961582769660140, 178.6962453788212031, -124.8244425039453915 ) ) ;
#9406=ORIENTED_EDGE ( 'NONE', *, *, #4346, .F. ) ;
#9409=ORIENTED_EDGE ( 'NONE', *, *, #4727, .T. ) ;
#9412=EDGE_CURVE ( 'NONE', #2975, #4344, #9993, .T. ) ;
#9416=VERTEX_POINT ( 'NONE', #9789 ) ;
#9423=DIRECTION ( 'NONE',  ( 0.9501779778103252028, 0.000000000000000000, 0.3117078928809489669 ) ) ;
#9425=EDGE_CURVE ( 'NONE', #569, #822, #11970, .T. ) ;
#9431=ORIENTED_EDGE ( 'NONE', *, *, #93, .F. ) ;
#9441=CARTESIAN_POINT ( 'NONE',  ( -19.98084489187587565, 177.8063731767314266, -125.5691280742910436 ) ) ;
#9450=CARTESIAN_POINT ( 'NONE',  ( 21.02276486677203593, 181.6974666944221042, -125.0994992711609370 ) ) ;
#9462=ORIENTED_EDGE ( 'NONE', *, *, #9087, .F. ) ;
#9466=DIRECTION ( 'NONE',  ( 0.3117078928809249860, -1.670400663243698742E-14, 0.9501779778103330854 ) ) ;
#9469=CARTESIAN_POINT ( 'NONE',  ( -19.98203294318189549, 182.6106388860948471, -125.5411158980709558 ) ) ;
#9498=CARTESIAN_POINT ( 'NONE',  ( 19.84263310680793069, 179.5276748199284214, -127.1852985703725807 ) ) ;
#9509=CARTESIAN_POINT ( 'NONE',  ( 19.98133380395517378, 177.8015904785984560, -125.5720248138883193 ) ) ;
#9517=CARTESIAN_POINT ( 'NONE',  ( 1.734723475976807094E-15, 180.2041921146324910, -179.7948474705909234 ) ) ;
#9518=DIRECTION ( 'NONE',  ( -1.000000000000000000, -1.186840563529527301E-16, 0.000000000000000000 ) ) ;
#9528=CARTESIAN_POINT ( 'NONE',  ( -20.00099490938537627, 182.7248142053001629, -124.9210440959558355 ) ) ;
#9547=ORIENTED_EDGE ( 'NONE', *, *, #2590, .F. ) ;
#9552=AXIS2_PLACEMENT_3D ( 'NONE', #6217, #585, #8816 ) ;
#9555=DIRECTION ( 'NONE',  ( -1.000000000000000000, 0.000000000000000000, 0.000000000000000000 ) ) ;
#9556=DIRECTION ( 'NONE',  ( -1.186840563529527301E-16, 1.000000000000000000, -0.000000000000000000 ) ) ;
#9559=CARTESIAN_POINT ( 'NONE',  ( -21.05708315573553691, 178.8782276755749194, -125.6123305554640837 ) ) ;
#9570=CARTESIAN_POINT ( 'NONE',  ( 4.335549520754014653E-15, 167.0000000000000000, -124.6807709998038405 ) ) ;
#9583=CARTESIAN_POINT ( 'NONE',  ( -19.99999999999999645, 177.7115707886035807, -124.6807709997916334 ) ) ;
#9607=ORIENTED_EDGE ( 'NONE', *, *, #3216, .T. ) ;
#9618=DIRECTION ( 'NONE',  ( -1.000000000000000000, 0.000000000000000000, 0.000000000000000000 ) ) ;
#9619=CARTESIAN_POINT ( 'NONE',  ( -21.06782237318494211, 179.3291273983845429, -126.1426500519474416 ) ) ;
#9620=ORIENTED_EDGE ( 'NONE', *, *, #5034, .F. ) ;
#9626=CARTESIAN_POINT ( 'NONE',  ( 4.335549520754014653E-15, 167.0000000000000000, -124.6807709998038405 ) ) ;
#9650=CARTESIAN_POINT ( 'NONE',  ( 19.99153366631225381, 178.9186500652280642, -123.8934111528711668 ) ) ;
#9668=CARTESIAN_POINT ( 'NONE',  ( -19.92945081678884023, 182.1752604789721488, -126.3669219011512297 ) ) ;
#9680=CARTESIAN_POINT ( 'NONE',  ( -19.98933286486646210, 178.9475762002984709, -125.5057985845799635 ) ) ;
#9687=CARTESIAN_POINT ( 'NONE',  ( -28.53314250459844459, 180.2041921146317236, -137.7978499286130898 ) ) ;
#9704=FACE_OUTER_BOUND ( 'NONE', #1057, .T. ) ;
#9711=CARTESIAN_POINT ( 'NONE',  ( 20.78030879612743931, 179.3744110069277724, -123.5640671919478280 ) ) ;
#9720=AXIS2_PLACEMENT_3D ( 'NONE', #7004, #11651, #10715 ) ;
#9723=CARTESIAN_POINT ( 'NONE',  ( -19.94418321653721549, 182.3098040923358951, -126.1872098885080646 ) ) ;
#9737=LINE ( 'NONE', #583, #213 ) ;
#9738=ORIENTED_EDGE ( 'NONE', *, *, #913, .F. ) ;
#9750=CARTESIAN_POINT ( 'NONE',  ( 4.454233577106967753E-15, 166.0000000000000000, -124.6807709998038405 ) ) ;
#9766=CARTESIAN_POINT ( 'NONE',  ( 20.73051967732101630, 180.6106195048880068, -123.3499684708650506 ) ) ;
#9783=CARTESIAN_POINT ( 'NONE',  ( -19.89470248115624074, 181.2369511437511278, -122.6240768797811853 ) ) ;
#9785=AXIS2_PLACEMENT_3D ( 'NONE', #4208, #4031, #1428 ) ;
#9789=CARTESIAN_POINT ( 'NONE',  ( 7.500000000000030198, -6.999999999999977796, -124.6807709998038405 ) ) ;
#9792=DIRECTION ( 'NONE',  ( -1.186840563529527301E-16, 1.000000000000000000, -0.000000000000000000 ) ) ;
#9799=ORIENTED_EDGE ( 'NONE', *, *, #11954, .T. ) ;
#9801=DIRECTION ( 'NONE',  ( -1.186840563529527301E-16, 1.000000000000000000, -0.000000000000000000 ) ) ;
#9805=AXIS2_PLACEMENT_3D ( 'NONE', #11169, #1774, #786 ) ;
#9806=CARTESIAN_POINT ( 'NONE',  ( 4.454233577106967753E-15, 166.0000000000000000, -124.6807709998038405 ) ) ;
#9811=DIRECTION ( 'NONE',  ( -0.9501779778103373042, 0.000000000000000000, 0.3117078928809121074 ) ) ;
#9812=CARTESIAN_POINT ( 'NONE',  ( -19.91081574664456610, 181.5182364730087272, -122.7941294590837913 ) ) ;
#9840=ORIENTED_EDGE ( 'NONE', *, *, #1645, .T. ) ;
#9842=CARTESIAN_POINT ( 'NONE',  ( 20.00056164720817264, 178.7050872343423578, -124.4636624667101472 ) ) ;
#9849=AXIS2_PLACEMENT_3D ( 'NONE', #4079, #8534, #10502 ) ;
#9851=VERTEX_POINT ( 'NONE', #5453 ) ;
#9852=ORIENTED_EDGE ( 'NONE', *, *, #8193, .T. ) ;
#9855=DIRECTION ( 'NONE',  ( 0.000000000000000000, -0.000000000000000000, -1.000000000000000000 ) ) ;
#9888=B_SPLINE_CURVE_WITH_KNOTS ( 'NONE', 3,
 ( #7010, #3135, #10798, #4130, #8929, #4074, #1348, #222, #3079, #10855, #460, #4256, #9928, #5980, #8024, #4185, #7905, #11553 ),
 .UNSPECIFIED., .F., .F.,
 ( 4, 2, 2, 2, 2, 2, 2, 2, 4 ),
 ( 0.002543027922241140014, 0.003172111293043450644, 0.003801194663845760841, 0.004430278034648071038, 0.005059361405450381668, 0.005688444776252692299, 0.006317528147055002929, 0.006946611517857312693, 0.007575694888659623323 ),
 .UNSPECIFIED. ) ;
#9893=DIRECTION ( 'NONE',  ( 0.000000000000000000, -1.757987137413040192E-14, 1.000000000000000000 ) ) ;
#9920=ORIENTED_EDGE ( 'NONE', *, *, #4202, .F. ) ;
#9926=CARTESIAN_POINT ( 'NONE',  ( -21.06782942783708634, 181.2569958439586912, -125.9973154456346407 ) ) ;
#9927=CARTESIAN_POINT ( 'NONE',  ( 21.06230101187101056, 180.1909031182395893, -126.4302698477766995 ) ) ;
#9928=CARTESIAN_POINT ( 'NONE',  ( 19.87222927861654043, 180.0711623112485711, -122.4236614295827081 ) ) ;
#9945=DIRECTION ( 'NONE',  ( -1.000000000000000000, 0.000000000000000000, 0.000000000000000000 ) ) ;
#9948=ORIENTED_EDGE ( 'NONE', *, *, #4342, .T. ) ;
#9953=CIRCLE ( 'NONE', #3842, 20.00000000000000000 ) ;
#9957=CARTESIAN_POINT ( 'NONE',  ( 1.734723475976807094E-15, 180.2041921146324910, -179.7948474705909234 ) ) ;
#9966=CARTESIAN_POINT ( 'NONE',  ( -20.75022707385176801, 180.8238523145130330, -123.4308975868758580 ) ) ;
#9971=FACE_OUTER_BOUND ( 'NONE', #6996, .T. ) ;
#9980=CARTESIAN_POINT ( 'NONE',  ( 8.500000000000007105, 167.0000000000000000, -124.6807709998038405 ) ) ;
#9992=CARTESIAN_POINT ( 'NONE',  ( -21.06346387521529806, 180.5375120120260135, -126.3982203091088508 ) ) ;
#9993=CIRCLE ( 'NONE', #4679, 1.500000000000000666 ) ;
#10007=FACE_OUTER_BOUND ( 'NONE', #4318, .T. ) ;
#10011=CARTESIAN_POINT ( 'NONE',  ( 19.87720992741833825, 179.7310258856144287, -122.4675742865357932 ) ) ;
#10012=CARTESIAN_POINT ( 'NONE',  ( -19.83216922734808207, 179.9533482554023180, -127.2663209614022293 ) ) ;
#10013=DIRECTION ( 'NONE',  ( 1.186840563529527301E-16, -1.000000000000000000, 0.000000000000000000 ) ) ;
#10019=AXIS2_PLACEMENT_3D ( 'NONE', #2551, #636, #8122 ) ;
#10028=CARTESIAN_POINT ( 'NONE',  ( -21.06507840625382499, 180.7491199079335047, -126.3364105811339329 ) ) ;
#10033=ADVANCED_FACE ( 'NONE', ( #5468 ), #3541, .T. ) ;
#10035=DIRECTION ( 'NONE',  ( 1.000000000000000000, 0.000000000000000000, 0.000000000000000000 ) ) ;
#10059=EDGE_LOOP ( 'NONE', ( #6133, #9852, #2415, #5485, #10514, #7105 ) ) ;
#10065=CARTESIAN_POINT ( 'NONE',  ( 19.94309760505412399, 182.0081148946152041, -123.1517843831254169 ) ) ;
#10086=EDGE_CURVE ( 'NONE', #2780, #6278, #5665, .T. ) ;
#10087=CARTESIAN_POINT ( 'NONE',  ( -21.06429661575627676, 179.7721861010548139, -126.3654905360901068 ) ) ;
#10090=DIRECTION ( 'NONE',  ( -1.000000000000000000, -1.156482317317870492E-16, 0.000000000000000000 ) ) ;
#10102=AXIS2_PLACEMENT_3D ( 'NONE', #2287, #6180, #9945 ) ;
#10116=CARTESIAN_POINT ( 'NONE',  ( -20.86426071607942845, 178.9745188154266771, -123.9720018873370009 ) ) ;
#10126=CARTESIAN_POINT ( 'NONE',  ( 19.98725040941994635, 181.3779265047164415, -125.6147582845246973 ) ) ;
#10128=VECTOR ( 'NONE', #7248, 1000.000000000000000 ) ;
#10147=TOROIDAL_SURFACE ( 'NONE', #9153, 19.00000000000000000, 1.000000000000000000 ) ;
#10162=CARTESIAN_POINT ( 'NONE',  ( 19.98390859781245510, 179.2016144824152093, -125.7887931655865685 ) ) ;
#10167=AXIS2_PLACEMENT_3D ( 'NONE', #3291, #9855, #9037 ) ;
#10179=( GEOMETRIC_REPRESENTATION_CONTEXT ( 3 ) GLOBAL_UNCERTAINTY_ASSIGNED_CONTEXT ( ( #1387 ) ) GLOBAL_UNIT_ASSIGNED_CONTEXT ( ( #8332, #6525, #7573 ) ) REPRESENTATION_CONTEXT ( 'NONE', 'WORKASPACE' ) );
#10193=CARTESIAN_POINT ( 'NONE',  ( 20.88840428458409448, 181.5134543962125804, -124.1041536322683783 ) ) ;
#10213=EDGE_LOOP ( 'NONE', ( #5411, #8177, #7633, #447 ) ) ;
#10215=CARTESIAN_POINT ( 'NONE',  ( -20.00000000000000000, 197.0000000000000000, -124.6807709998038405 ) ) ;
#10227=CARTESIAN_POINT ( 'NONE',  ( 19.98507655485050094, 179.1352618259597307, -125.7279253762596483 ) ) ;
#10243=CARTESIAN_POINT ( 'NONE',  ( 21.06656027035116807, 179.5228220458012629, -126.2633464264420695 ) ) ;
#10245=AXIS2_PLACEMENT_3D ( 'NONE', #9570, #6041, #4007 ) ;
#10247=CARTESIAN_POINT ( 'NONE',  ( -19.98529084832767566, 177.9024039722029613, -123.8679874905754161 ) ) ;
#10251=ORIENTED_EDGE ( 'NONE', *, *, #307, .T. ) ;
#10257=CARTESIAN_POINT ( 'NONE',  ( -20.77482174596494247, 180.9926187296578348, -123.5402880645763730 ) ) ;
#10258=CARTESIAN_POINT ( 'NONE',  ( 21.05508193123089100, 181.5508406828318471, -125.5707457972380325 ) ) ;
#10265=CARTESIAN_POINT ( 'NONE',  ( 21.06306891294164529, 179.9350108970479596, -126.4083702064951211 ) ) ;
#10270=VERTEX_POINT ( 'NONE', #8994 ) ;
#10286=CARTESIAN_POINT ( 'NONE',  ( 19.97135992617064915, 177.8754454934489218, -125.7601421070351222 ) ) ;
#10288=CARTESIAN_POINT ( 'NONE',  ( 6.500000000000030198, -6.999999999999977796, -124.6807709998038405 ) ) ;
#10301=DIRECTION ( 'NONE',  ( 0.000000000000000000, 1.632680918566399772E-14, -1.000000000000000000 ) ) ;
#10302=CARTESIAN_POINT ( 'NONE',  ( -20.98196205190248875, 178.7079620517401963, -124.7263650620788269 ) ) ;
#10303=FACE_OUTER_BOUND ( 'NONE', #2598, .T. ) ;
#10313=CARTESIAN_POINT ( 'NONE',  ( 19.97825765123714348, 180.7277658390849808, -126.0785619755266822 ) ) ;
#10316=DIRECTION ( 'NONE',  ( -0.3117078928809153826, -1.979053562451413181E-14, -0.9501779778103363050 ) ) ;
#10321=CARTESIAN_POINT ( 'NONE',  ( 4.454233577106967753E-15, 166.0000000000000000, -124.6807709998038405 ) ) ;
#10360=CARTESIAN_POINT ( 'NONE',  ( 19.83206362640841647, 180.0177979251707825, -127.2672250451624905 ) ) ;
#10417=VERTEX_POINT ( 'NONE', #5331 ) ;
#10427=CIRCLE ( 'NONE', #3126, 1.000000000000000888 ) ;
#10428=ORIENTED_EDGE ( 'NONE', *, *, #9425, .F. ) ;
#10431=ORIENTED_EDGE ( 'NONE', *, *, #1258, .F. ) ;
#10437=CARTESIAN_POINT ( 'NONE',  ( 21.00606259948788335, 181.7116910486332984, -124.9297615680210498 ) ) ;
#10442=CARTESIAN_POINT ( 'NONE',  ( -7.500000000000000888, 166.0000000000000000, -124.6807709998038405 ) ) ;
#10460=CARTESIAN_POINT ( 'NONE',  ( -20.92339290342903979, 181.6071613487999059, -124.3124672736065577 ) ) ;
#10463=ORIENTED_EDGE ( 'NONE', *, *, #8356, .T. ) ;
#10485=EDGE_CURVE ( 'NONE', #2611, #9028, #6626, .T. ) ;
#10489=CARTESIAN_POINT ( 'NONE',  ( -19.99365627236732834, 178.8147210300960239, -125.2696703636239448 ) ) ;
#10502=DIRECTION ( 'NONE',  ( -1.000000000000000000, 0.000000000000000000, 0.000000000000000000 ) ) ;
#10509=DIRECTION ( 'NONE',  ( -1.000000000000000000, 0.000000000000000000, 0.000000000000000000 ) ) ;
#10514=ORIENTED_EDGE ( 'NONE', *, *, #4342, .F. ) ;
#10515=VECTOR ( 'NONE', #10958, 1000.000000000000000 ) ;
#10544=CARTESIAN_POINT ( 'NONE',  ( -19.99638601442813979, 178.7511098637216946, -125.0988180456752161 ) ) ;
#10565=TOROIDAL_SURFACE ( 'NONE', #12159, 19.00000000000000000, 1.000000000000000000 ) ;
#10566=CARTESIAN_POINT ( 'NONE',  ( 13.32222501832767847, 180.2041921146325762, -184.1652315311843893 ) ) ;
#10568=AXIS2_PLACEMENT_3D ( 'NONE', #3145, #8773, #1413 ) ;
#10586=ORIENTED_EDGE ( 'NONE', *, *, #4727, .F. ) ;
#10608=CARTESIAN_POINT ( 'NONE',  ( -19.99604380743649301, 177.7113426136561998, -125.1086484215899191 ) ) ;
#10611=ORIENTED_EDGE ( 'NONE', *, *, #3726, .F. ) ;
#10623=CARTESIAN_POINT ( 'NONE',  ( 20.72709806565185531, 179.8688360349001414, -123.3353893985419774 ) ) ;
#10635=ADVANCED_FACE ( 'NONE', ( #9235 ), #5671, .T. ) ;
#10638=CARTESIAN_POINT ( 'NONE',  ( 19.91452063025001706, 178.8212236027263202, -122.8311025665217073 ) ) ;
#10651=TOROIDAL_SURFACE ( 'NONE', #5313, 10.00000000000003730, 1.499999999999998002 ) ;
#10652=CARTESIAN_POINT ( 'NONE',  ( -19.90963648991972690, 178.8974959161414233, -122.7794448225913584 ) ) ;
#10665=CARTESIAN_POINT ( 'NONE',  ( -19.97123502809169793, 177.8744193083314826, -125.7706088136690852 ) ) ;
#10669=ORIENTED_EDGE ( 'NONE', *, *, #1692, .T. ) ;
#10680=CARTESIAN_POINT ( 'NONE',  ( 21.06824446939009121, 179.1652731564143721, -126.0114239279031807 ) ) ;
#10705=EDGE_LOOP ( 'NONE', ( #11680, #8078, #7488, #3115, #7736, #5302 ) ) ;
#10713=APPLICATION_CONTEXT ( 'automotive_design' ) ;
#10715=DIRECTION ( 'NONE',  ( 1.000000000000000000, 1.186840563529527301E-16, 0.000000000000000000 ) ) ;
#10723=AXIS2_PLACEMENT_3D ( 'NONE', #9957, #10945, #5134 ) ;
#10729=AXIS2_PLACEMENT_3D ( 'NONE', #12211, #5651, #9423 ) ;
#10766=CIRCLE ( 'NONE', #10568, 20.00000000000000000 ) ;
#10775=LINE ( 'NONE', #11771, #10515 ) ;
#10788=CARTESIAN_POINT ( 'NONE',  ( -19.99537293950516670, 177.7157818389469242, -125.1249387510345912 ) ) ;
#10789=ORIENTED_EDGE ( 'NONE', *, *, #6134, .T. ) ;
#10797=CARTESIAN_POINT ( 'NONE',  ( 19.83679575339899159, 180.6775276936280079, -127.2308936265927315 ) ) ;
#10798=CARTESIAN_POINT ( 'NONE',  ( 19.99669161722127697, 177.7723063827659473, -124.2664439125946103 ) ) ;
#10799=DIRECTION ( 'NONE',  ( -1.186840563529527301E-16, 1.000000000000000000, -0.000000000000000000 ) ) ;
#10825=CIRCLE ( 'NONE', #7070, 1.499999999999998224 ) ;
#10829=CARTESIAN_POINT ( 'NONE',  ( 20.00073208655986079, 178.6939288504570129, -124.5619098010894277 ) ) ;
#10843=CARTESIAN_POINT ( 'NONE',  ( -19.99906152404484061, 177.7018673789226568, -124.9038452892194329 ) ) ;
#10849=ORIENTED_EDGE ( 'NONE', *, *, #6928, .F. ) ;
#10853=CARTESIAN_POINT ( 'NONE',  ( 19.91813571189143417, 181.6502384987539926, -122.8703185013854409 ) ) ;
#10855=CARTESIAN_POINT ( 'NONE',  ( 19.89204199682034258, 179.2535526226286606, -122.6034008110078304 ) ) ;
#10868=CARTESIAN_POINT ( 'NONE',  ( 19.87433925290471848, 179.8947790015472208, -122.4423054685512113 ) ) ;
#10884=CARTESIAN_POINT ( 'NONE',  ( 19.98584444751550393, 177.8987813746903441, -123.9137298384522836 ) ) ;
#10885=AXIS2_PLACEMENT_3D ( 'NONE', #8779, #236, #6120 ) ;
#10886=CARTESIAN_POINT ( 'NONE',  ( -19.87519864879852349, 178.8871479037923393, -126.9115732480538838 ) ) ;
#10898=ADVANCED_FACE ( 'NONE', ( #1323 ), #770, .F. ) ;
#10903=FACE_OUTER_BOUND ( 'NONE', #7900, .T. ) ;
#10904=DIRECTION ( 'NONE',  ( 0.000000000000000000, 0.000000000000000000, 1.000000000000000000 ) ) ;
#10908=B_SPLINE_CURVE_WITH_KNOTS ( 'NONE', 3,
 ( #804, #9262, #12113, #3624, #7412, #6483, #1853, #2841, #3761, #9450, #10437, #1978, #4415, #8189, #8913, #6143 ),
 .UNSPECIFIED., .F., .F.,
 ( 4, 2, 2, 2, 2, 2, 2, 4 ),
 ( 0.0009136864633593878935, 0.001421019263031339909, 0.001928352062703291925, 0.002435684862375243724, 0.002943017662047195740, 0.003450350461719148623, 0.003957683261391099772, 0.004972348860735044569 ),
 .UNSPECIFIED. ) ;
#10915=CARTESIAN_POINT ( 'NONE',  ( -21.06624625262745099, 181.3699762841097538, -125.8703140475546149 ) ) ;
#10919=CARTESIAN_POINT ( 'NONE',  ( -19.95147628160284370, 182.1113810128487387, -123.2819571381896822 ) ) ;
#10920=TOROIDAL_SURFACE ( 'NONE', #5600, 6.500000000000005329, 1.000000000000000000 ) ;
#10927=EDGE_CURVE ( 'NONE', #20, #12185, #5017, .T. ) ;
#10930=DIRECTION ( 'NONE',  ( -1.000000000000000000, 0.000000000000000000, 0.000000000000000000 ) ) ;
#10936=CARTESIAN_POINT ( 'NONE',  ( 20.72575232321667116, 179.9202923768740732, -123.3302915314655479 ) ) ;
#10938=CARTESIAN_POINT ( 'NONE',  ( -19.87412339327474342, 180.5265370758251606, -122.4403904965001288 ) ) ;
#10945=DIRECTION ( 'NONE',  ( -0.000000000000000000, -1.000000000000000000, -1.757987137413040192E-14 ) ) ;
#10954=CARTESIAN_POINT ( 'NONE',  ( -21.06231667407016772, 180.1636738665369251, -126.4297697749043010 ) ) ;
#10958=DIRECTION ( 'NONE',  ( -1.186840563529527301E-16, 1.000000000000000000, -0.000000000000000000 ) ) ;
#10967=DIRECTION ( 'NONE',  ( -1.000000000000000000, 0.000000000000000000, 0.000000000000000000 ) ) ;
#10968=CARTESIAN_POINT ( 'NONE',  ( 8.937118865183852088E-16, 196.0000000000000000, -124.6807709998038405 ) ) ;
#10972=DIRECTION ( 'NONE',  ( -1.186840563529527301E-16, 1.000000000000000000, -0.000000000000000000 ) ) ;
#10979=CARTESIAN_POINT ( 'NONE',  ( -20.77482174596494247, 180.9926187296578348, -123.5402880645763730 ) ) ;
#10994=CARTESIAN_POINT ( 'NONE',  ( 19.98378750576280538, 182.6226996931179087, -125.4995243108248388 ) ) ;
#10996=VECTOR ( 'NONE', #9466, 1000.000000000000000 ) ;
#10998=CARTESIAN_POINT ( 'NONE',  ( -19.94337906914356395, 178.3983333771979858, -123.1706592317244144 ) ) ;
#11011=CARTESIAN_POINT ( 'NONE',  ( 19.83177985141341892, 179.9887880572465519, -127.2693050255385714 ) ) ;
#11023=FACE_OUTER_BOUND ( 'NONE', #7332, .T. ) ;
#11032=CARTESIAN_POINT ( 'NONE',  ( -20.77322673479996951, 179.4133438526717441, -123.5311657466897373 ) ) ;
#11044=CARTESIAN_POINT ( 'NONE',  ( -19.95913600371365959, 180.2478989036688972, -123.1890436974040313 ) ) ;
#11046=ADVANCED_FACE ( 'NONE', ( #1161 ), #3994, .T. ) ;
#11051=DIRECTION ( 'NONE',  ( -0.3117078928809425831, -5.319854888938806247E-14, 0.9501779778103273122 ) ) ;
#11056=CARTESIAN_POINT ( 'NONE',  ( 20.96297238888044845, 181.6803933783718890, -124.5802004042857334 ) ) ;
#11060=EDGE_CURVE ( 'NONE', #8373, #569, #6013, .T. ) ;
#11076=ORIENTED_EDGE ( 'NONE', *, *, #11060, .F. ) ;
#11088=CIRCLE ( 'NONE', #2016, 8.500000000000035527 ) ;
#11090=CARTESIAN_POINT ( 'NONE',  ( 19.98182870893229079, 179.3422780683628162, -125.8969293818015984 ) ) ;
#11093=DIRECTION ( 'NONE',  ( 0.000000000000000000, 1.788286221017408824E-14, -1.000000000000000000 ) ) ;
#11105=CARTESIAN_POINT ( 'NONE',  ( 21.06333566525091072, 179.8959387247087705, -126.3976994828154545 ) ) ;
#11109=CARTESIAN_POINT ( 'NONE',  ( -19.99085265605563677, 178.9337235835365050, -123.8700625655956173 ) ) ;
#11119=CARTESIAN_POINT ( 'NONE',  ( 7.750278301654327006E-16, 197.0000000000000000, -124.6807709998038405 ) ) ;
#11122=CARTESIAN_POINT ( 'NONE',  ( 19.98950317961507750, 182.6598950331495814, -125.3472100544021686 ) ) ;
#11142=CARTESIAN_POINT ( 'NONE',  ( 20.89973826391392464, 178.8616761932901795, -124.1694459372093178 ) ) ;
#11146=CARTESIAN_POINT ( 'NONE',  ( -19.83893667468079869, 179.6461197167075170, -127.2139938056598965 ) ) ;
#11147=AXIS2_PLACEMENT_3D ( 'NONE', #8698, #11599, #9555 ) ;
#11156=CARTESIAN_POINT ( 'NONE',  ( 19.89196810756490663, 178.6505532842396633, -126.7594064012678388 ) ) ;
#11169=CARTESIAN_POINT ( 'NONE',  ( 7.750278301654327006E-16, 197.0000000000000000, -124.6807709998038405 ) ) ;
#11172=DIRECTION ( 'NONE',  ( -1.000000000000000000, -1.186840563529527301E-16, 0.000000000000000000 ) ) ;
#11173=CARTESIAN_POINT ( 'NONE',  ( 21.06244748020267465, 180.0923556010718869, -126.4260852699257356 ) ) ;
#11178=CARTESIAN_POINT ( 'NONE',  ( -20.73637609554099726, 179.7535993509491163, -123.3744064433501677 ) ) ;
#11180=ORIENTED_EDGE ( 'NONE', *, *, #3885, .T. ) ;
#11186=ORIENTED_EDGE ( 'NONE', *, *, #1007, .T. ) ;
#11191=CARTESIAN_POINT ( 'NONE',  ( 19.99966070409250207, 182.7093770945723463, -124.8756968753967271 ) ) ;
#11197=CARTESIAN_POINT ( 'NONE',  ( -29.95840947131392795, 180.2041921146317236, -138.2654117679345802 ) ) ;
#11203=VERTEX_POINT ( 'NONE', #3870 ) ;
#11212=CARTESIAN_POINT ( 'NONE',  ( -19.96713961980339391, 182.4999670356679076, -125.8362662571105517 ) ) ;
#11235=FILL_AREA_STYLE ('',( #7450 ) ) ;
#11245=CARTESIAN_POINT ( 'NONE',  ( -20.74457341359024198, 179.6607161185452810, -123.4086842481865602 ) ) ;
#11254=CARTESIAN_POINT ( 'NONE',  ( 19.98725602524029554, 182.5262326453932076, -123.9529870253308133 ) ) ;
#11267=CARTESIAN_POINT ( 'NONE',  ( 19.90078111156755014, 181.8690955493196384, -126.6770338381014938 ) ) ;
#11287=CIRCLE ( 'NONE', #27, 1.499999999999999112 ) ;
#11291=CARTESIAN_POINT ( 'NONE',  ( -19.03136272649511085, 180.2041921146316668, -134.6807709998038547 ) ) ;
#11292=CARTESIAN_POINT ( 'NONE',  ( -20.71964524312745937, 180.2041921146310415, -123.3053720114591272 ) ) ;
#11299=DIRECTION ( 'NONE',  ( 0.000000000000000000, 1.689469820081754479E-14, -1.000000000000000000 ) ) ;
#11301=AXIS2_PLACEMENT_3D ( 'NONE', #8319, #6511, #4473 ) ;
#11302=EDGE_CURVE ( 'NONE', #1954, #10270, #2260, .T. ) ;
#11310=TOROIDAL_SURFACE ( 'NONE', #5978, 8.500000000000003553, 1.000000000000000000 ) ;
#11312=EDGE_CURVE ( 'NONE', #7974, #2536, #6998, .T. ) ;
#11330=CYLINDRICAL_SURFACE ( 'NONE', #4398, 1.500000000000000444 ) ;
#11350=CARTESIAN_POINT ( 'NONE',  ( 19.98008256664037674, 179.4972950632025857, -125.9865773177933477 ) ) ;
#11354=CARTESIAN_POINT ( 'NONE',  ( -19.99764744648923909, 178.7270483677477841, -125.0101186568579266 ) ) ;
#11357=ORIENTED_EDGE ( 'NONE', *, *, #10927, .F. ) ;
#11362=DIRECTION ( 'NONE',  ( -0.000000000000000000, -1.000000000000000000, -1.757987137413040192E-14 ) ) ;
#11375=EDGE_CURVE ( 'NONE', #8373, #1329, #3854, .T. ) ;
#11378=CARTESIAN_POINT ( 'NONE',  ( -19.97506881502268428, 181.0839254472395510, -123.4722291287969114 ) ) ;
#11383=CARTESIAN_POINT ( 'NONE',  ( 19.90629981715767016, 178.9629118261667600, -122.7457835946827913 ) ) ;
#11384=CARTESIAN_POINT ( 'NONE',  ( -21.06303090563296365, 181.4372473149129803, -125.7691643379808255 ) ) ;
#11405=ORIENTED_EDGE ( 'NONE', *, *, #10485, .T. ) ;
#11407=SURFACE_STYLE_FILL_AREA ( #11235 ) ;
#11439=AXIS2_PLACEMENT_3D ( 'NONE', #9517, #936, #4709 ) ;
#11445=CARTESIAN_POINT ( 'NONE',  ( 19.98289417481194974, 179.1164216503652540, -123.6441077975231480 ) ) ;
#11447=CARTESIAN_POINT ( 'NONE',  ( -19.99909886256255476, 181.7106308440128544, -124.9041157096212800 ) ) ;
#11473=EDGE_LOOP ( 'NONE', ( #9738, #3562, #6130, #1283 ) ) ;
#11479=DIRECTION ( 'NONE',  ( -1.000000000000000000, 0.000000000000000000, 0.000000000000000000 ) ) ;
#11497=ORIENTED_EDGE ( 'NONE', *, *, #5846, .T. ) ;
#11528=FACE_OUTER_BOUND ( 'NONE', #2048, .T. ) ;
#11531=SHAPE_DEFINITION_REPRESENTATION ( #1126, #12068 ) ;
#11544=CIRCLE ( 'NONE', #2257, 11.50000000000001066 ) ;
#11547=AXIS2_PLACEMENT_3D ( 'NONE', #4913, #3008, #2948 ) ;
#11553=CARTESIAN_POINT ( 'NONE',  ( 19.90865200055593220, 181.4799304009739558, -122.7714319726113104 ) ) ;
#11560=DIRECTION ( 'NONE',  ( -0.3117078928809153826, -1.979053562451413181E-14, -0.9501779778103363050 ) ) ;
#11578=PRODUCT_DEFINITION_FORMATION_WITH_SPECIFIED_SOURCE ( 'ANY', '', #12175, .NOT_KNOWN. ) ;
#11588=CARTESIAN_POINT ( 'NONE',  ( -19.83523559361558242, 180.6327028742894640, -127.2433017073463759 ) ) ;
#11599=DIRECTION ( 'NONE',  ( -1.186840563529527301E-16, 1.000000000000000000, -0.000000000000000000 ) ) ;
#11605=DIRECTION ( 'NONE',  ( -1.186840563529527301E-16, 1.000000000000000000, -0.000000000000000000 ) ) ;
#11621=CARTESIAN_POINT ( 'NONE',  ( -19.97946249231785032, 182.4386859306654856, -123.7598397378640556 ) ) ;
#11625=CARTESIAN_POINT ( 'NONE',  ( 20.84205126700888400, 179.0243517598608776, -123.8490133567502340 ) ) ;
#11651=DIRECTION ( 'NONE',  ( 1.186840563529527301E-16, -1.000000000000000000, 0.000000000000000000 ) ) ;
#11667=EDGE_CURVE ( 'NONE', #7054, #5440, #8968, .T. ) ;
#11668=ORIENTED_EDGE ( 'NONE', *, *, #8586, .F. ) ;
#11672=VERTEX_POINT ( 'NONE', #4527 ) ;
#11679=CARTESIAN_POINT ( 'NONE',  ( 20.77382952161539720, 179.4090627415999961, -123.5337882278526251 ) ) ;
#11680=ORIENTED_EDGE ( 'NONE', *, *, #2747, .F. ) ;
#11738=CARTESIAN_POINT ( 'NONE',  ( -20.00000000000000000, 182.6968134406616002, -124.6807709998189466 ) ) ;
#11742=CARTESIAN_POINT ( 'NONE',  ( 21.02894813693603382, 178.6886507591858049, -125.1318251072521832 ) ) ;
#11750=CARTESIAN_POINT ( 'NONE',  ( 21.06240745282767435, 180.2041921146315246, -126.4269926335259413 ) ) ;
#11752=CARTESIAN_POINT ( 'NONE',  ( 19.95943535220619580, 180.3310120364355953, -123.1936495657158019 ) ) ;
#11771=CARTESIAN_POINT ( 'NONE',  ( 7.500000000000006217, 197.0000000000000000, -124.6807709998038405 ) ) ;
#11784=DIRECTION ( 'NONE',  ( 0.3117078928809249860, -1.670400663243698742E-14, 0.9501779778103330854 ) ) ;
#11789=FACE_OUTER_BOUND ( 'NONE', #3900, .T. ) ;
#11790=CARTESIAN_POINT ( 'NONE',  ( -21.02406183884818347, 181.6953053563225353, -125.1140174421107929 ) ) ;
#11794=DIRECTION ( 'NONE',  ( 1.186840563529527301E-16, -1.000000000000000000, 0.000000000000000000 ) ) ;
#11809=CARTESIAN_POINT ( 'NONE',  ( 20.73848121498308572, 179.7277624624672399, -123.3832113358915876 ) ) ;
#11810=AXIS2_PLACEMENT_3D ( 'NONE', #4625, #8207, #4431 ) ;
#11838=EDGE_CURVE ( 'NONE', #2536, #7974, #10766, .T. ) ;
#11839=AXIS2_PLACEMENT_3D ( 'NONE', #9316, #1841, #10301 ) ;
#11845=CARTESIAN_POINT ( 'NONE',  ( -21.06817635203014305, 179.2720927603041332, -126.1063812806455218 ) ) ;
#11864=CARTESIAN_POINT ( 'NONE',  ( -19.91081574664456610, 181.5182364730087272, -122.7941294590837913 ) ) ;
#11865=FACE_OUTER_BOUND ( 'NONE', #1482, .T. ) ;
#11880=CARTESIAN_POINT ( 'NONE',  ( -19.84982438750066081, 181.1124051037951119, -127.1282150172683458 ) ) ;
#11882=ORIENTED_EDGE ( 'NONE', *, *, #4181, .F. ) ;
#11895=EDGE_LOOP ( 'NONE', ( #7639, #971, #9920, #5290 ) ) ;
#11923=CARTESIAN_POINT ( 'NONE',  ( 20.97617298093462779, 181.6955223378353992, -124.6801735093379477 ) ) ;
#11926=CARTESIAN_POINT ( 'NONE',  ( -19.88356468709224956, 179.4771400433740780, -122.5253713362719594 ) ) ;
#11933=AXIS2_PLACEMENT_3D ( 'NONE', #10968, #6273, #12158 ) ;
#11936=DIRECTION ( 'NONE',  ( -1.186840563529527301E-16, 1.000000000000000000, -0.000000000000000000 ) ) ;
#11943=CARTESIAN_POINT ( 'NONE',  ( -19.86685153722994457, 181.4191362699532704, -126.9922420271958288 ) ) ;
#11944=EDGE_LOOP ( 'NONE', ( #7617, #8544, #3575, #4590 ) ) ;
#11954=EDGE_CURVE ( 'NONE', #9851, #559, #1299, .T. ) ;
#11957=AXIS2_PLACEMENT_3D ( 'NONE', #9048, #10904, #7955 ) ;
#11970=CIRCLE ( 'NONE', #9204, 0.9999999999999991118 ) ;
#11973=CARTESIAN_POINT ( 'NONE',  ( -19.90421694283016407, 179.0016913079787173, -122.7245617132216040 ) ) ;
#11985=CARTESIAN_POINT ( 'NONE',  ( 19.99429366071382930, 181.6100965659588553, -125.2310411471055716 ) ) ;
#12005=CARTESIAN_POINT ( 'NONE',  ( 7.750278301654327992E-16, 197.0000000000000000, -124.6807709998038405 ) ) ;
#12010=CARTESIAN_POINT ( 'NONE',  ( 20.71964524312746647, 180.2041921146487766, -123.3053720114591414 ) ) ;
#12019=CARTESIAN_POINT ( 'NONE',  ( 7.500000000000008882, 166.0000000000000000, -124.6807709998038405 ) ) ;
#12020=EDGE_CURVE ( 'NONE', #11203, #2536, #5425, .T. ) ;
#12035=CARTESIAN_POINT ( 'NONE',  ( -20.72047049683759212, 180.3431580008786170, -123.3086960613613172 ) ) ;
#12048=CARTESIAN_POINT ( 'NONE',  ( 21.06742223667033542, 181.2647206388604673, -125.9812270727733789 ) ) ;
#12062=CARTESIAN_POINT ( 'NONE',  ( 20.86632180319404029, 178.9255784920988503, -127.0464874675043205 ) ) ;
#12067=CARTESIAN_POINT ( 'NONE',  ( -20.74379340896704704, 180.7482559160401365, -123.4054388444186827 ) ) ;
#12068=SHAPE_REPRESENTATION ( 'Forming Shoe Axle Center Pin', ( #11957 ), #3662 ) ;
#12074=CARTESIAN_POINT ( 'NONE',  ( -19.92844181622918143, 182.1616102128938621, -126.3751434161658409 ) ) ;
#12075=LINE ( 'NONE', #3583, #7984 ) ;
#12078=CARTESIAN_POINT ( 'NONE',  ( 20.00000000000000355, 177.7115707886026144, -124.6807709998038547 ) ) ;
#12079=MANIFOLD_SOLID_BREP ( 'Fillet9', #2753 ) ;
#12082=ORIENTED_EDGE ( 'NONE', *, *, #2368, .T. ) ;
#12104=CARTESIAN_POINT ( 'NONE',  ( -19.91230007514456446, 178.8584202414884601, -122.8074605759933888 ) ) ;
#12113=CARTESIAN_POINT ( 'NONE',  ( 21.06348120957193260, 180.5399482493916139, -126.3977753017352370 ) ) ;
#12117=CARTESIAN_POINT ( 'NONE',  ( 21.06758144644436115, 180.9571029733192233, -126.2348846925512049 ) ) ;
#12127=CARTESIAN_POINT ( 'NONE',  ( 20.00000000000000000, 182.6968134406613160, -124.6807709998155076 ) ) ;
#12130=CARTESIAN_POINT ( 'NONE',  ( 19.00000000000000000, 196.0000000000000000, -124.6807709998038405 ) ) ;
#12139=TOROIDAL_SURFACE ( 'NONE', #6794, 19.00000000000000000, 1.000000000000000000 ) ;
#12154=CARTESIAN_POINT ( 'NONE',  ( 19.91278132667089906, 178.4073888321768209, -126.5495299892900647 ) ) ;
#12158=DIRECTION ( 'NONE',  ( 1.000000000000000000, 0.000000000000000000, 0.000000000000000000 ) ) ;
#12159=AXIS2_PLACEMENT_3D ( 'NONE', #4896, #8060, #3467 ) ;
#12167=CARTESIAN_POINT ( 'NONE',  ( -29.95840947131394572, 180.2041921146317236, -138.2654117679345234 ) ) ;
#12172=CARTESIAN_POINT ( 'NONE',  ( -19.97571278480728196, 179.3030001708650332, -123.4829212133057865 ) ) ;
#12173=CARTESIAN_POINT ( 'NONE',  ( 4.216865464401061553E-15, 168.0000000000000000, -124.6807709998038405 ) ) ;
#12175=PRODUCT ( 'Forming Shoe Axle Center Pin', 'Forming Shoe Axle Center Pin', '', ( #8750 ) ) ;
#12179=ORIENTED_EDGE ( 'NONE', *, *, #3216, .F. ) ;
#12183=CARTESIAN_POINT ( 'NONE',  ( 21.02964448618781645, 181.6776138650130292, -125.1863404894149880 ) ) ;
#12185=VERTEX_POINT ( 'NONE', #4152 ) ;
#12188=LINE ( 'NONE', #11197, #5113 ) ;
#12191=EDGE_CURVE ( 'NONE', #2139, #9220, #2479, .T. ) ;
#12202=CARTESIAN_POINT ( 'NONE',  ( -20.89267889318610472, 181.5262592919334566, -124.1284379062907703 ) ) ;
#12211=CARTESIAN_POINT ( 'NONE',  ( -28.53314250459844459, 180.2041921146317236, -137.7978499286130898 ) ) ;
#12232=ORIENTED_EDGE ( 'NONE', *, *, #6134, .F. ) ;
#12236=ORIENTED_EDGE ( 'NONE', *, *, #7002, .F. ) ;
ENDSEC;
END-ISO-10303-21;
